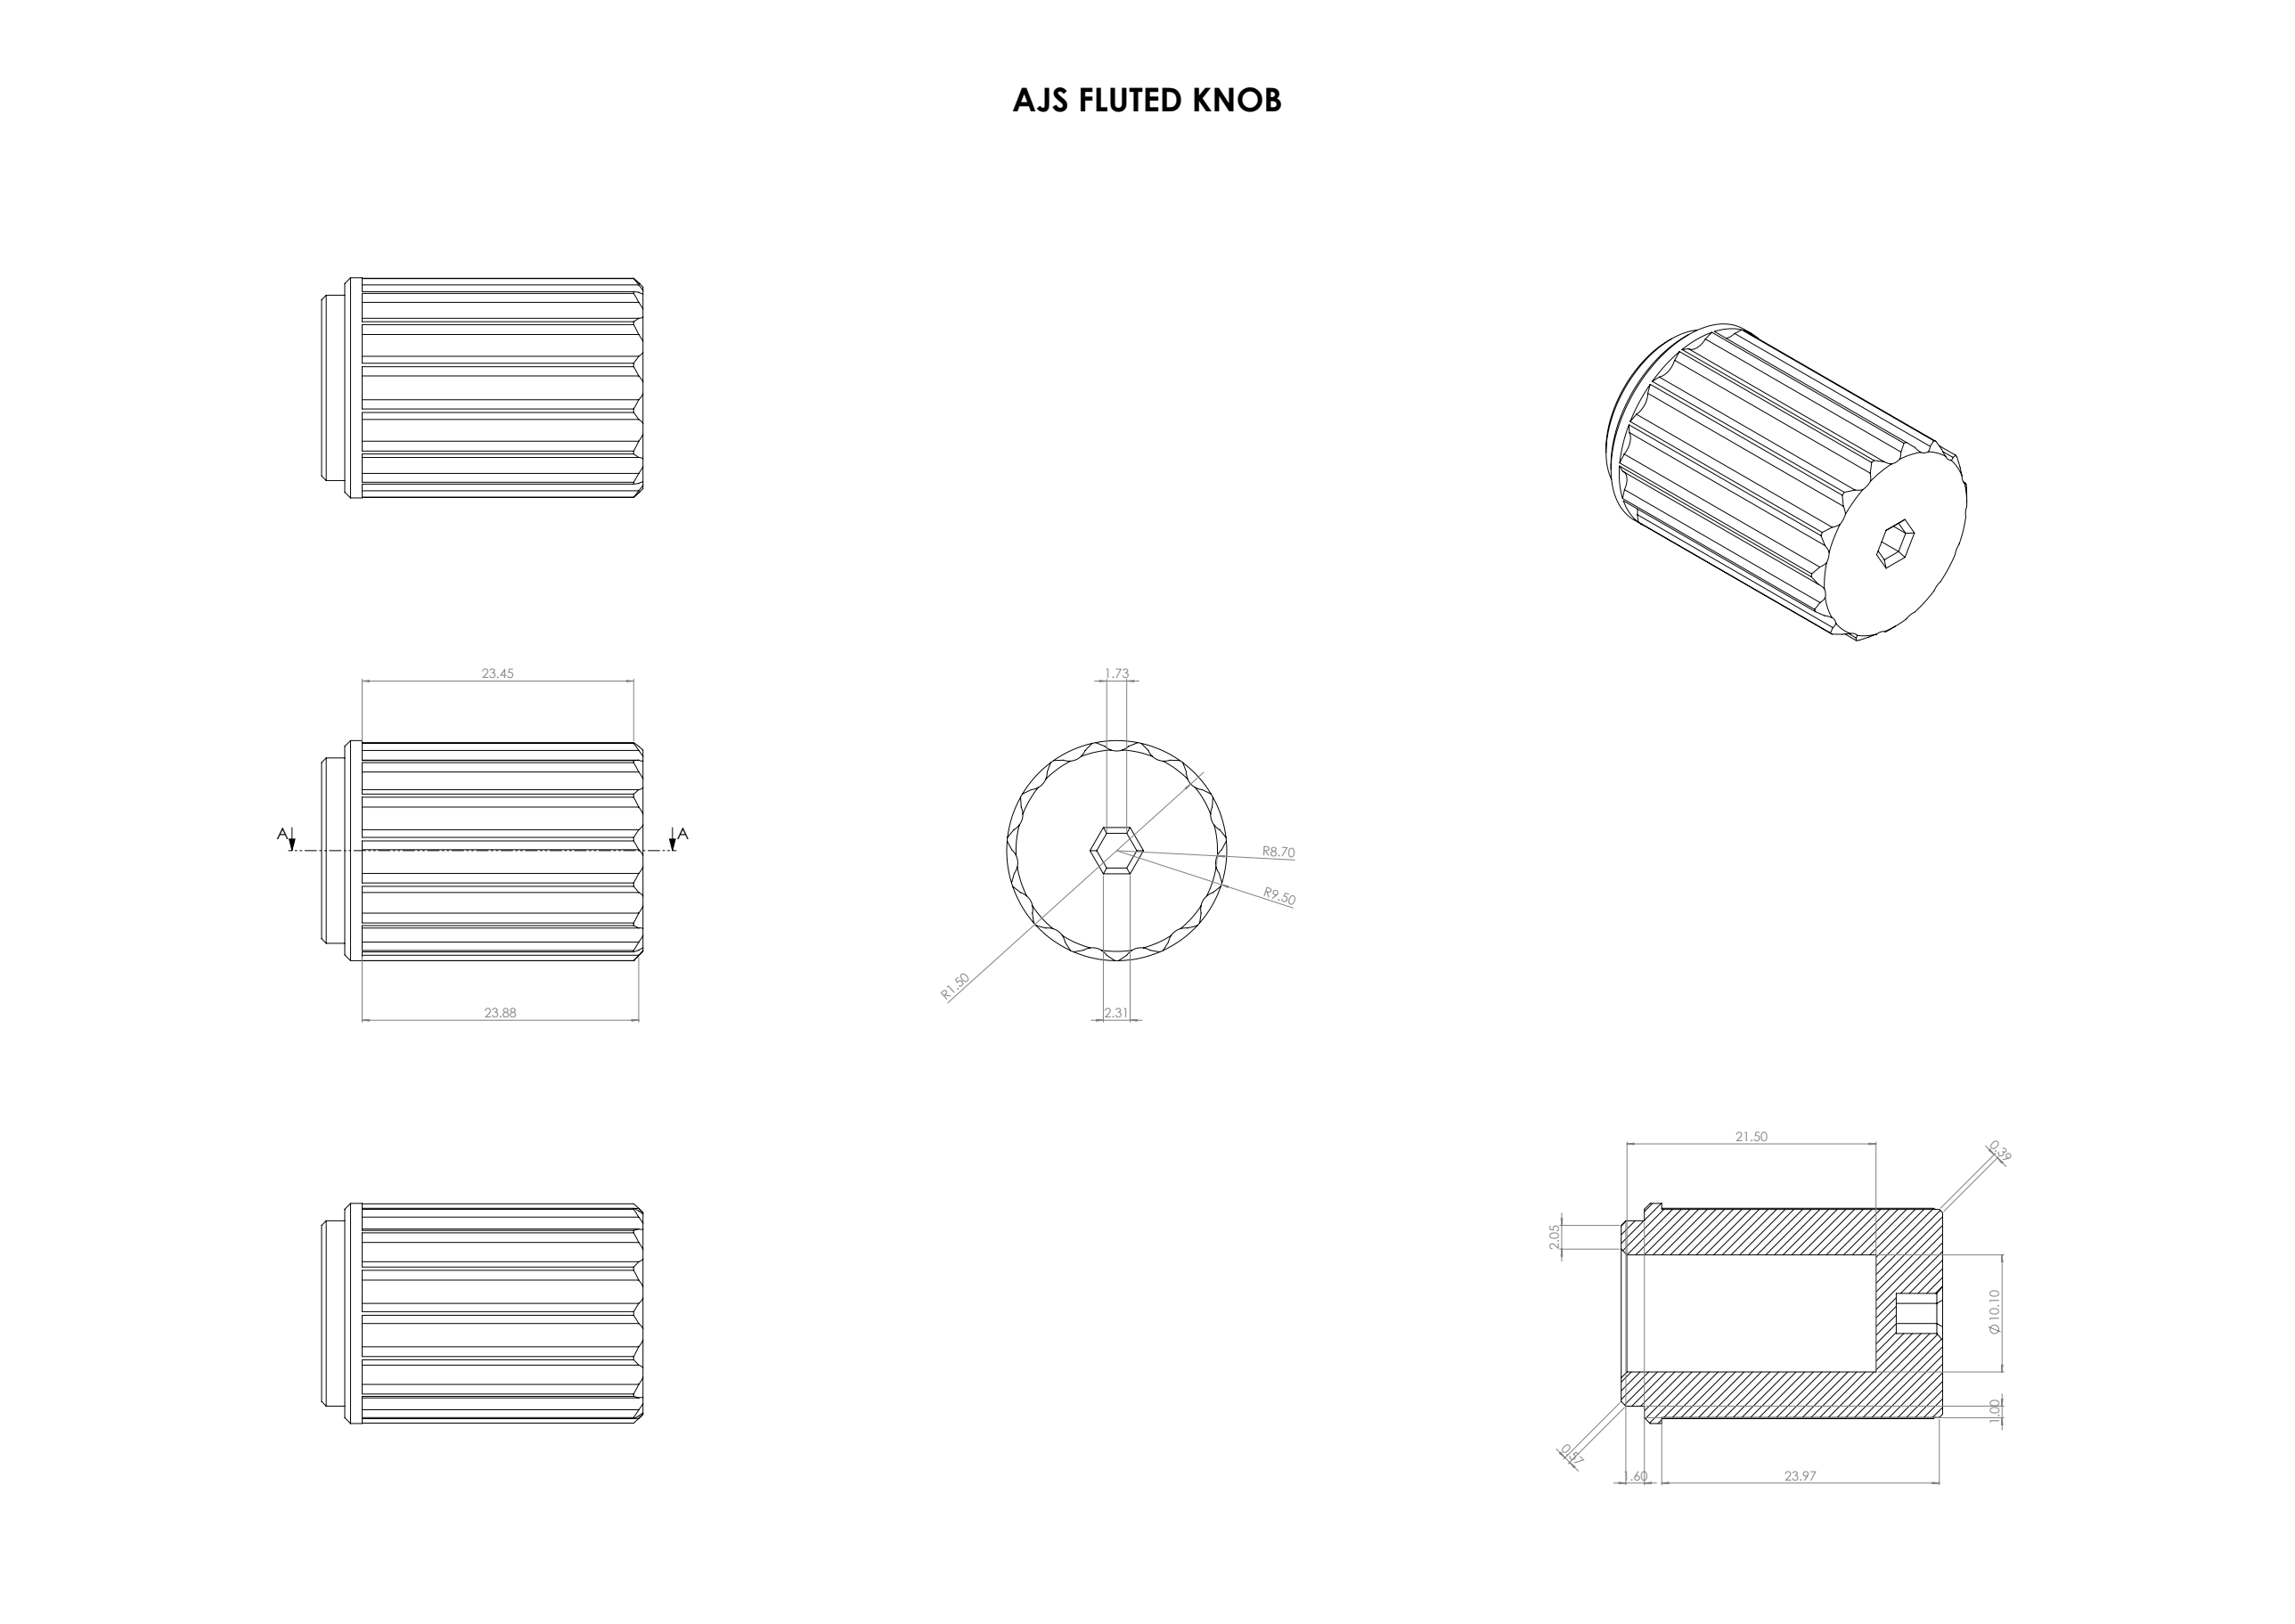
ISO-10303-21;
HEADER;
/* Generated by software containing ST-Developer
 * from STEP Tools, Inc. (www.steptools.com) 
 */

FILE_DESCRIPTION(
/* description */ (''),
/* implementation_level */ '2;1');

FILE_NAME(
/* name */ '06_AJS_Fluted_Knob.step',
/* time_stamp */ '2026-10-21T01:56:51-07:00',
/* author */ (''),
/* organization */ (''),
/* preprocessor_version */ 'ST-DEVELOPER v20.2',
/* originating_system */ 'Autodesk Translation Framework v15.15.0.0',
/* authorisation */ '');

FILE_SCHEMA (('AUTOMOTIVE_DESIGN { 1 0 10303 214 3 1 1 }'));
ENDSEC;

DATA;
#10=MECHANICAL_DESIGN_GEOMETRIC_PRESENTATION_REPRESENTATION('',(#287),#82384);
#202=(
BOUNDED_CURVE()
B_SPLINE_CURVE(2,(#80282,#80283,#80284),.UNSPECIFIED.,.F.,.F.)
B_SPLINE_CURVE_WITH_KNOTS((3,3),(0.095709435566232,0.188213402372322),
 .UNSPECIFIED.)
CURVE()
GEOMETRIC_REPRESENTATION_ITEM()
RATIONAL_B_SPLINE_CURVE((1.00220608042206,1.00217204690889,1.00001144171476))
REPRESENTATION_ITEM('')
);
#203=(
BOUNDED_CURVE()
B_SPLINE_CURVE(2,(#80312,#80313,#80314),.UNSPECIFIED.,.F.,.F.)
B_SPLINE_CURVE_WITH_KNOTS((3,3),(0.000244613971281809,0.0927485807773717),
 .UNSPECIFIED.)
CURVE()
GEOMETRIC_REPRESENTATION_ITEM()
RATIONAL_B_SPLINE_CURVE((1.00001144171476,1.00217204690889,1.00220608042206))
REPRESENTATION_ITEM('')
);
#204=(
BOUNDED_CURVE()
B_SPLINE_CURVE(2,(#80322,#80323,#80324),.UNSPECIFIED.,.F.,.F.)
B_SPLINE_CURVE_WITH_KNOTS((3,3),(0.0957094355662357,0.188213402372324),
 .UNSPECIFIED.)
CURVE()
GEOMETRIC_REPRESENTATION_ITEM()
RATIONAL_B_SPLINE_CURVE((1.00220608042216,1.00217204690899,1.00001144171476))
REPRESENTATION_ITEM('')
);
#205=(
BOUNDED_CURVE()
B_SPLINE_CURVE(2,(#80469,#80470,#80471),.UNSPECIFIED.,.F.,.F.)
B_SPLINE_CURVE_WITH_KNOTS((3,3),(0.000244613971281676,0.0927485807773712),
 .UNSPECIFIED.)
CURVE()
GEOMETRIC_REPRESENTATION_ITEM()
RATIONAL_B_SPLINE_CURVE((1.00001144171476,1.00217204690889,1.00220608042206))
REPRESENTATION_ITEM('')
);
#206=(
BOUNDED_CURVE()
B_SPLINE_CURVE(2,(#80475,#80476,#80477),.UNSPECIFIED.,.F.,.F.)
B_SPLINE_CURVE_WITH_KNOTS((3,3),(0.0957094355662342,0.188213402372322),
 .UNSPECIFIED.)
CURVE()
GEOMETRIC_REPRESENTATION_ITEM()
RATIONAL_B_SPLINE_CURVE((1.00220608042205,1.00217204690887,1.00001144171476))
REPRESENTATION_ITEM('')
);
#207=(
BOUNDED_CURVE()
B_SPLINE_CURVE(2,(#80504,#80505,#80506),.UNSPECIFIED.,.F.,.F.)
B_SPLINE_CURVE_WITH_KNOTS((3,3),(0.000244613971281263,0.0927485807773676),
 .UNSPECIFIED.)
CURVE()
GEOMETRIC_REPRESENTATION_ITEM()
RATIONAL_B_SPLINE_CURVE((1.00001144171476,1.00217204690908,1.00220608042225))
REPRESENTATION_ITEM('')
);
#208=(
BOUNDED_CURVE()
B_SPLINE_CURVE(2,(#80510,#80511,#80512),.UNSPECIFIED.,.F.,.F.)
B_SPLINE_CURVE_WITH_KNOTS((3,3),(0.0957094355662345,0.188213402372322),
 .UNSPECIFIED.)
CURVE()
GEOMETRIC_REPRESENTATION_ITEM()
RATIONAL_B_SPLINE_CURVE((1.00220608042216,1.00217204690899,1.00001144171476))
REPRESENTATION_ITEM('')
);
#209=(
BOUNDED_CURVE()
B_SPLINE_CURVE(2,(#80539,#80540,#80541),.UNSPECIFIED.,.F.,.F.)
B_SPLINE_CURVE_WITH_KNOTS((3,3),(0.000244613971281759,0.0927485807773703),
 .UNSPECIFIED.)
CURVE()
GEOMETRIC_REPRESENTATION_ITEM()
RATIONAL_B_SPLINE_CURVE((1.00001144171476,1.00217204690897,1.00220608042214))
REPRESENTATION_ITEM('')
);
#210=(
BOUNDED_CURVE()
B_SPLINE_CURVE(2,(#80545,#80546,#80547),.UNSPECIFIED.,.F.,.F.)
B_SPLINE_CURVE_WITH_KNOTS((3,3),(0.0957094355662337,0.188213402372321),
 .UNSPECIFIED.)
CURVE()
GEOMETRIC_REPRESENTATION_ITEM()
RATIONAL_B_SPLINE_CURVE((1.00220608042215,1.00217204690897,1.00001144171476))
REPRESENTATION_ITEM('')
);
#211=(
BOUNDED_CURVE()
B_SPLINE_CURVE(2,(#80574,#80575,#80576),.UNSPECIFIED.,.F.,.F.)
B_SPLINE_CURVE_WITH_KNOTS((3,3),(0.000244613971281829,0.0927485807773718),
 .UNSPECIFIED.)
CURVE()
GEOMETRIC_REPRESENTATION_ITEM()
RATIONAL_B_SPLINE_CURVE((1.00001144171476,1.00217204690888,1.00220608042205))
REPRESENTATION_ITEM('')
);
#212=(
BOUNDED_CURVE()
B_SPLINE_CURVE(2,(#80580,#80581,#80582),.UNSPECIFIED.,.F.,.F.)
B_SPLINE_CURVE_WITH_KNOTS((3,3),(0.0957094355662314,0.188213402372321),
 .UNSPECIFIED.)
CURVE()
GEOMETRIC_REPRESENTATION_ITEM()
RATIONAL_B_SPLINE_CURVE((1.00220608042206,1.00217204690889,1.00001144171476))
REPRESENTATION_ITEM('')
);
#213=(
BOUNDED_CURVE()
B_SPLINE_CURVE(2,(#80609,#80610,#80611),.UNSPECIFIED.,.F.,.F.)
B_SPLINE_CURVE_WITH_KNOTS((3,3),(0.000244613971281268,0.0927485807773693),
 .UNSPECIFIED.)
CURVE()
GEOMETRIC_REPRESENTATION_ITEM()
RATIONAL_B_SPLINE_CURVE((1.00001144171476,1.00217204690897,1.00220608042215))
REPRESENTATION_ITEM('')
);
#214=(
BOUNDED_CURVE()
B_SPLINE_CURVE(2,(#80615,#80616,#80617),.UNSPECIFIED.,.F.,.F.)
B_SPLINE_CURVE_WITH_KNOTS((3,3),(0.0957094355662326,0.188213402372321),
 .UNSPECIFIED.)
CURVE()
GEOMETRIC_REPRESENTATION_ITEM()
RATIONAL_B_SPLINE_CURVE((1.00220608042217,1.002172046909,1.00001144171476))
REPRESENTATION_ITEM('')
);
#215=(
BOUNDED_CURVE()
B_SPLINE_CURVE(2,(#80644,#80645,#80646),.UNSPECIFIED.,.F.,.F.)
B_SPLINE_CURVE_WITH_KNOTS((3,3),(0.000244613971283097,0.0927485807773713),
 .UNSPECIFIED.)
CURVE()
GEOMETRIC_REPRESENTATION_ITEM()
RATIONAL_B_SPLINE_CURVE((1.00001144171476,1.002172046909,1.00220608042218))
REPRESENTATION_ITEM('')
);
#216=(
BOUNDED_CURVE()
B_SPLINE_CURVE(2,(#80650,#80651,#80652),.UNSPECIFIED.,.F.,.F.)
B_SPLINE_CURVE_WITH_KNOTS((3,3),(0.0957094355662316,0.188213402372321),
 .UNSPECIFIED.)
CURVE()
GEOMETRIC_REPRESENTATION_ITEM()
RATIONAL_B_SPLINE_CURVE((1.00220608042227,1.00217204690909,1.00001144171476))
REPRESENTATION_ITEM('')
);
#217=(
BOUNDED_CURVE()
B_SPLINE_CURVE(2,(#80679,#80680,#80681),.UNSPECIFIED.,.F.,.F.)
B_SPLINE_CURVE_WITH_KNOTS((3,3),(0.000244613971281759,0.09274858077737),
 .UNSPECIFIED.)
CURVE()
GEOMETRIC_REPRESENTATION_ITEM()
RATIONAL_B_SPLINE_CURVE((1.00001144171476,1.00217204690888,1.00220608042205))
REPRESENTATION_ITEM('')
);
#218=(
BOUNDED_CURVE()
B_SPLINE_CURVE(2,(#80685,#80686,#80687),.UNSPECIFIED.,.F.,.F.)
B_SPLINE_CURVE_WITH_KNOTS((3,3),(0.0957094355662316,0.18821340237232),
 .UNSPECIFIED.)
CURVE()
GEOMETRIC_REPRESENTATION_ITEM()
RATIONAL_B_SPLINE_CURVE((1.00220608042213,1.00217204690896,1.00001144171476))
REPRESENTATION_ITEM('')
);
#219=(
BOUNDED_CURVE()
B_SPLINE_CURVE(2,(#80714,#80715,#80716),.UNSPECIFIED.,.F.,.F.)
B_SPLINE_CURVE_WITH_KNOTS((3,3),(0.000244613971281648,0.0927485807773707),
 .UNSPECIFIED.)
CURVE()
GEOMETRIC_REPRESENTATION_ITEM()
RATIONAL_B_SPLINE_CURVE((1.00001144171476,1.00217204690889,1.00220608042206))
REPRESENTATION_ITEM('')
);
#220=(
BOUNDED_CURVE()
B_SPLINE_CURVE(2,(#80720,#80721,#80722),.UNSPECIFIED.,.F.,.F.)
B_SPLINE_CURVE_WITH_KNOTS((3,3),(0.0957094355662329,0.188213402372321),
 .UNSPECIFIED.)
CURVE()
GEOMETRIC_REPRESENTATION_ITEM()
RATIONAL_B_SPLINE_CURVE((1.00220608042214,1.00217204690897,1.00001144171476))
REPRESENTATION_ITEM('')
);
#221=(
BOUNDED_CURVE()
B_SPLINE_CURVE(2,(#80749,#80750,#80751),.UNSPECIFIED.,.F.,.F.)
B_SPLINE_CURVE_WITH_KNOTS((3,3),(0.000244613971281549,0.0927485807773708),
 .UNSPECIFIED.)
CURVE()
GEOMETRIC_REPRESENTATION_ITEM()
RATIONAL_B_SPLINE_CURVE((1.00001144171476,1.002172046909,1.00220608042218))
REPRESENTATION_ITEM('')
);
#222=(
BOUNDED_CURVE()
B_SPLINE_CURVE(2,(#80755,#80756,#80757),.UNSPECIFIED.,.F.,.F.)
B_SPLINE_CURVE_WITH_KNOTS((3,3),(0.0957094355662331,0.188213402372322),
 .UNSPECIFIED.)
CURVE()
GEOMETRIC_REPRESENTATION_ITEM()
RATIONAL_B_SPLINE_CURVE((1.00220608042225,1.00217204690908,1.00001144171476))
REPRESENTATION_ITEM('')
);
#223=(
BOUNDED_CURVE()
B_SPLINE_CURVE(2,(#80784,#80785,#80786),.UNSPECIFIED.,.F.,.F.)
B_SPLINE_CURVE_WITH_KNOTS((3,3),(0.000244613971281458,0.0927485807773696),
 .UNSPECIFIED.)
CURVE()
GEOMETRIC_REPRESENTATION_ITEM()
RATIONAL_B_SPLINE_CURVE((1.00001144171476,1.00217204690908,1.00220608042225))
REPRESENTATION_ITEM('')
);
#224=(
BOUNDED_CURVE()
B_SPLINE_CURVE(2,(#80790,#80791,#80792),.UNSPECIFIED.,.F.,.F.)
B_SPLINE_CURVE_WITH_KNOTS((3,3),(0.0957094355662337,0.188213402372322),
 .UNSPECIFIED.)
CURVE()
GEOMETRIC_REPRESENTATION_ITEM()
RATIONAL_B_SPLINE_CURVE((1.00220608042226,1.00217204690909,1.00001144171476))
REPRESENTATION_ITEM('')
);
#225=(
BOUNDED_CURVE()
B_SPLINE_CURVE(2,(#80819,#80820,#80821),.UNSPECIFIED.,.F.,.F.)
B_SPLINE_CURVE_WITH_KNOTS((3,3),(0.000244613971281769,0.0927485807773717),
 .UNSPECIFIED.)
CURVE()
GEOMETRIC_REPRESENTATION_ITEM()
RATIONAL_B_SPLINE_CURVE((1.00001144171476,1.00217204690888,1.00220608042205))
REPRESENTATION_ITEM('')
);
#226=(
BOUNDED_CURVE()
B_SPLINE_CURVE(2,(#80825,#80826,#80827),.UNSPECIFIED.,.F.,.F.)
B_SPLINE_CURVE_WITH_KNOTS((3,3),(0.0957094355662335,0.188213402372321),
 .UNSPECIFIED.)
CURVE()
GEOMETRIC_REPRESENTATION_ITEM()
RATIONAL_B_SPLINE_CURVE((1.00220608042207,1.0021720469089,1.00001144171476))
REPRESENTATION_ITEM('')
);
#227=(
BOUNDED_CURVE()
B_SPLINE_CURVE(2,(#80854,#80855,#80856),.UNSPECIFIED.,.F.,.F.)
B_SPLINE_CURVE_WITH_KNOTS((3,3),(0.00024461397128167,0.0927485807773707),
 .UNSPECIFIED.)
CURVE()
GEOMETRIC_REPRESENTATION_ITEM()
RATIONAL_B_SPLINE_CURVE((1.00001144171476,1.00217204690889,1.00220608042207))
REPRESENTATION_ITEM('')
);
#228=(
BOUNDED_CURVE()
B_SPLINE_CURVE(2,(#80860,#80861,#80862),.UNSPECIFIED.,.F.,.F.)
B_SPLINE_CURVE_WITH_KNOTS((3,3),(0.0957094355662347,0.188213402372323),
 .UNSPECIFIED.)
CURVE()
GEOMETRIC_REPRESENTATION_ITEM()
RATIONAL_B_SPLINE_CURVE((1.00220608042226,1.00217204690908,1.00001144171476))
REPRESENTATION_ITEM('')
);
#229=(
BOUNDED_CURVE()
B_SPLINE_CURVE(2,(#80889,#80890,#80891),.UNSPECIFIED.,.F.,.F.)
B_SPLINE_CURVE_WITH_KNOTS((3,3),(0.000244613971281467,0.0927485807773707),
 .UNSPECIFIED.)
CURVE()
GEOMETRIC_REPRESENTATION_ITEM()
RATIONAL_B_SPLINE_CURVE((1.00001144171476,1.00217204690889,1.00220608042206))
REPRESENTATION_ITEM('')
);
#230=(
BOUNDED_CURVE()
B_SPLINE_CURVE(2,(#80895,#80896,#80897),.UNSPECIFIED.,.F.,.F.)
B_SPLINE_CURVE_WITH_KNOTS((3,3),(0.0957094355662333,0.188213402372321),
 .UNSPECIFIED.)
CURVE()
GEOMETRIC_REPRESENTATION_ITEM()
RATIONAL_B_SPLINE_CURVE((1.00220608042207,1.00217204690889,1.00001144171476))
REPRESENTATION_ITEM('')
);
#231=(
BOUNDED_CURVE()
B_SPLINE_CURVE(2,(#80924,#80925,#80926),.UNSPECIFIED.,.F.,.F.)
B_SPLINE_CURVE_WITH_KNOTS((3,3),(0.000244613971281619,0.0927485807773719),
 .UNSPECIFIED.)
CURVE()
GEOMETRIC_REPRESENTATION_ITEM()
RATIONAL_B_SPLINE_CURVE((1.00001144171476,1.00217204690898,1.00220608042215))
REPRESENTATION_ITEM('')
);
#249=SHAPE_REPRESENTATION_RELATIONSHIP('SRR','None',#82483,#268);
#268=ADVANCED_BREP_SHAPE_REPRESENTATION('',(#306),#82382);
#287=STYLED_ITEM('',(#82624),#306);
#306=MANIFOLD_SOLID_BREP('Body1',#30678);
#1003=CYLINDRICAL_SURFACE('',#33159,5.05);
#1004=CYLINDRICAL_SURFACE('',#33164,1.5);
#1005=CYLINDRICAL_SURFACE('',#33171,9.5);
#1006=CYLINDRICAL_SURFACE('',#33204,1.5);
#1007=CYLINDRICAL_SURFACE('',#33211,1.5);
#1008=CYLINDRICAL_SURFACE('',#33218,1.5);
#1009=CYLINDRICAL_SURFACE('',#33225,1.5);
#1010=CYLINDRICAL_SURFACE('',#33232,1.5);
#1011=CYLINDRICAL_SURFACE('',#33239,1.5);
#1012=CYLINDRICAL_SURFACE('',#33246,1.5);
#1013=CYLINDRICAL_SURFACE('',#33253,1.5);
#1014=CYLINDRICAL_SURFACE('',#33260,1.5);
#1015=CYLINDRICAL_SURFACE('',#33267,1.5);
#1016=CYLINDRICAL_SURFACE('',#33274,1.5);
#1017=CYLINDRICAL_SURFACE('',#33281,1.5);
#1018=CYLINDRICAL_SURFACE('',#33288,1.5);
#1019=CYLINDRICAL_SURFACE('',#33295,1.5);
#1020=CYLINDRICAL_SURFACE('',#33332,8.);
#1777=CIRCLE('',#33156,5.55);
#1778=CIRCLE('',#33157,5.05);
#1779=CIRCLE('',#33158,5.05);
#1780=CIRCLE('',#33160,5.05);
#1781=CIRCLE('',#33162,7.6);
#1782=CIRCLE('',#33165,1.5);
#1783=CIRCLE('',#33166,1.5);
#1784=CIRCLE('',#33169,9.5);
#1785=CIRCLE('',#33170,8.7);
#1786=CIRCLE('',#33172,9.5);
#1787=CIRCLE('',#33173,9.5);
#1788=CIRCLE('',#33174,9.5);
#1789=CIRCLE('',#33175,9.5);
#1790=CIRCLE('',#33176,9.5);
#1791=CIRCLE('',#33177,9.5);
#1792=CIRCLE('',#33178,9.5);
#1793=CIRCLE('',#33179,9.5);
#1794=CIRCLE('',#33180,9.5);
#1795=CIRCLE('',#33181,9.5);
#1796=CIRCLE('',#33182,9.5);
#1797=CIRCLE('',#33183,9.5);
#1798=CIRCLE('',#33184,9.5);
#1799=CIRCLE('',#33185,9.5);
#1800=CIRCLE('',#33186,9.5);
#1801=CIRCLE('',#33187,9.5);
#1802=CIRCLE('',#33188,9.5);
#1803=CIRCLE('',#33189,9.5);
#1804=CIRCLE('',#33190,9.5);
#1805=CIRCLE('',#33191,9.5);
#1806=CIRCLE('',#33192,9.5);
#1807=CIRCLE('',#33193,9.5);
#1808=CIRCLE('',#33194,9.5);
#1809=CIRCLE('',#33195,9.5);
#1810=CIRCLE('',#33196,9.5);
#1811=CIRCLE('',#33197,9.5);
#1812=CIRCLE('',#33198,9.5);
#1813=CIRCLE('',#33199,9.5);
#1814=CIRCLE('',#33200,9.5);
#1815=CIRCLE('',#33201,9.5);
#1816=CIRCLE('',#33202,9.5);
#1817=CIRCLE('',#33205,1.5);
#1818=CIRCLE('',#33206,1.5);
#1819=CIRCLE('',#33209,8.7);
#1820=CIRCLE('',#33212,1.5);
#1821=CIRCLE('',#33213,1.5);
#1822=CIRCLE('',#33216,8.7);
#1823=CIRCLE('',#33219,1.5);
#1824=CIRCLE('',#33220,1.5);
#1825=CIRCLE('',#33223,8.7);
#1826=CIRCLE('',#33226,1.5);
#1827=CIRCLE('',#33227,1.5);
#1828=CIRCLE('',#33230,8.7);
#1829=CIRCLE('',#33233,1.5);
#1830=CIRCLE('',#33234,1.5);
#1831=CIRCLE('',#33237,8.7);
#1832=CIRCLE('',#33240,1.5);
#1833=CIRCLE('',#33241,1.5);
#1834=CIRCLE('',#33244,8.7);
#1835=CIRCLE('',#33247,1.5);
#1836=CIRCLE('',#33248,1.5);
#1837=CIRCLE('',#33251,8.7);
#1838=CIRCLE('',#33254,1.5);
#1839=CIRCLE('',#33255,1.5);
#1840=CIRCLE('',#33258,8.7);
#1841=CIRCLE('',#33261,1.5);
#1842=CIRCLE('',#33262,1.5);
#1843=CIRCLE('',#33265,8.7);
#1844=CIRCLE('',#33268,1.5);
#1845=CIRCLE('',#33269,1.5);
#1846=CIRCLE('',#33272,8.7);
#1847=CIRCLE('',#33275,1.5);
#1848=CIRCLE('',#33276,1.5);
#1849=CIRCLE('',#33279,8.7);
#1850=CIRCLE('',#33282,1.5);
#1851=CIRCLE('',#33283,1.5);
#1852=CIRCLE('',#33286,8.7);
#1853=CIRCLE('',#33289,1.5);
#1854=CIRCLE('',#33290,1.5);
#1855=CIRCLE('',#33293,8.7);
#1856=CIRCLE('',#33296,1.5);
#1857=CIRCLE('',#33297,1.5);
#1858=CIRCLE('',#33309,8.7);
#1859=CIRCLE('',#33331,8.);
#1860=CIRCLE('',#33333,8.);
#1861=CIRCLE('',#33335,9.);
#2063=CONICAL_SURFACE('',#33155,5.3,0.785398163397451);
#2064=CONICAL_SURFACE('',#33168,9.1,0.785398163397454);
#2065=CONICAL_SURFACE('',#33208,9.1,0.785398163397454);
#2066=CONICAL_SURFACE('',#33215,9.1,0.785398163397454);
#2067=CONICAL_SURFACE('',#33222,9.1,0.785398163397454);
#2068=CONICAL_SURFACE('',#33229,9.1,0.785398163397454);
#2069=CONICAL_SURFACE('',#33236,9.1,0.785398163397454);
#2070=CONICAL_SURFACE('',#33243,9.1,0.785398163397454);
#2071=CONICAL_SURFACE('',#33250,9.1,0.785398163397454);
#2072=CONICAL_SURFACE('',#33257,9.1,0.785398163397454);
#2073=CONICAL_SURFACE('',#33264,9.1,0.785398163397454);
#2074=CONICAL_SURFACE('',#33271,9.1,0.785398163397454);
#2075=CONICAL_SURFACE('',#33278,9.1,0.785398163397454);
#2076=CONICAL_SURFACE('',#33285,9.1,0.785398163397454);
#2077=CONICAL_SURFACE('',#33292,9.1,0.785398163397454);
#2078=CONICAL_SURFACE('',#33329,9.1,0.785398163397454);
#2079=CONICAL_SURFACE('',#33330,7.8,0.785398163397454);
#2080=CONICAL_SURFACE('',#33336,9.25,0.785398163397445);
#3220=B_SPLINE_CURVE_WITH_KNOTS('',3,(#80296,#80297,#80298,#80299,#80300,
#80301),.UNSPECIFIED.,.F.,.F.,(4,2,4),(0.300223039487565,0.349769627099692,
0.370274237441758),.UNSPECIFIED.);
#3221=B_SPLINE_CURVE_WITH_KNOTS('',3,(#80304,#80305,#80306,#80307,#80308,
#80309),.UNSPECIFIED.,.F.,.F.,(4,2,4),(0.128903119732732,0.149407730074798,
0.198954317686925),.UNSPECIFIED.);
#3222=B_SPLINE_CURVE_WITH_KNOTS('',3,(#80326,#80327,#80328,#80329,#80330,
#80331),.UNSPECIFIED.,.F.,.F.,(4,2,4),(0.128903119732731,0.149407730074798,
0.198954317686925),.UNSPECIFIED.);
#3223=B_SPLINE_CURVE_WITH_KNOTS('',3,(#80461,#80462,#80463,#80464,#80465,
#80466),.UNSPECIFIED.,.F.,.F.,(4,2,4),(0.300223039487565,0.349769627099692,
0.370274237441758),.UNSPECIFIED.);
#3224=B_SPLINE_CURVE_WITH_KNOTS('',3,(#80479,#80480,#80481,#80482,#80483,
#80484),.UNSPECIFIED.,.F.,.F.,(4,2,4),(0.128903119732732,0.149407730074798,
0.198954317686925),.UNSPECIFIED.);
#3225=B_SPLINE_CURVE_WITH_KNOTS('',3,(#80496,#80497,#80498,#80499,#80500,
#80501),.UNSPECIFIED.,.F.,.F.,(4,2,4),(0.300223039487565,0.349769627099692,
0.370274237441758),.UNSPECIFIED.);
#3226=B_SPLINE_CURVE_WITH_KNOTS('',3,(#80514,#80515,#80516,#80517,#80518,
#80519),.UNSPECIFIED.,.F.,.F.,(4,2,4),(0.128903119732732,0.149407730074798,
0.198954317686925),.UNSPECIFIED.);
#3227=B_SPLINE_CURVE_WITH_KNOTS('',3,(#80531,#80532,#80533,#80534,#80535,
#80536),.UNSPECIFIED.,.F.,.F.,(4,2,4),(0.300223039487565,0.349769627099692,
0.370274237441758),.UNSPECIFIED.);
#3228=B_SPLINE_CURVE_WITH_KNOTS('',3,(#80549,#80550,#80551,#80552,#80553,
#80554),.UNSPECIFIED.,.F.,.F.,(4,2,4),(0.128903119732731,0.149407730074798,
0.198954317686925),.UNSPECIFIED.);
#3229=B_SPLINE_CURVE_WITH_KNOTS('',3,(#80566,#80567,#80568,#80569,#80570,
#80571),.UNSPECIFIED.,.F.,.F.,(4,2,4),(0.300223039487565,0.349769627099692,
0.370274237441758),.UNSPECIFIED.);
#3230=B_SPLINE_CURVE_WITH_KNOTS('',3,(#80584,#80585,#80586,#80587,#80588,
#80589),.UNSPECIFIED.,.F.,.F.,(4,2,4),(0.128903119732732,0.149407730074798,
0.198954317686925),.UNSPECIFIED.);
#3231=B_SPLINE_CURVE_WITH_KNOTS('',3,(#80601,#80602,#80603,#80604,#80605,
#80606),.UNSPECIFIED.,.F.,.F.,(4,2,4),(0.300223039487565,0.349769627099692,
0.370274237441759),.UNSPECIFIED.);
#3232=B_SPLINE_CURVE_WITH_KNOTS('',3,(#80619,#80620,#80621,#80622,#80623,
#80624),.UNSPECIFIED.,.F.,.F.,(4,2,4),(0.128903119732732,0.149407730074798,
0.198954317686923),.UNSPECIFIED.);
#3233=B_SPLINE_CURVE_WITH_KNOTS('',3,(#80636,#80637,#80638,#80639,#80640,
#80641),.UNSPECIFIED.,.F.,.F.,(4,2,4),(0.300223039487567,0.349769627099692,
0.370274237441759),.UNSPECIFIED.);
#3234=B_SPLINE_CURVE_WITH_KNOTS('',3,(#80654,#80655,#80656,#80657,#80658,
#80659),.UNSPECIFIED.,.F.,.F.,(4,2,4),(0.128903119732731,0.149407730074798,
0.198954317686924),.UNSPECIFIED.);
#3235=B_SPLINE_CURVE_WITH_KNOTS('',3,(#80671,#80672,#80673,#80674,#80675,
#80676),.UNSPECIFIED.,.F.,.F.,(4,2,4),(0.300223039487565,0.349769627099692,
0.370274237441758),.UNSPECIFIED.);
#3236=B_SPLINE_CURVE_WITH_KNOTS('',3,(#80689,#80690,#80691,#80692,#80693,
#80694),.UNSPECIFIED.,.F.,.F.,(4,2,4),(0.128903119732731,0.149407730074798,
0.198954317686925),.UNSPECIFIED.);
#3237=B_SPLINE_CURVE_WITH_KNOTS('',3,(#80706,#80707,#80708,#80709,#80710,
#80711),.UNSPECIFIED.,.F.,.F.,(4,2,4),(0.300223039487565,0.349769627099692,
0.370274237441758),.UNSPECIFIED.);
#3238=B_SPLINE_CURVE_WITH_KNOTS('',3,(#80724,#80725,#80726,#80727,#80728,
#80729),.UNSPECIFIED.,.F.,.F.,(4,2,4),(0.128903119732732,0.149407730074798,
0.198954317686924),.UNSPECIFIED.);
#3239=B_SPLINE_CURVE_WITH_KNOTS('',3,(#80741,#80742,#80743,#80744,#80745,
#80746),.UNSPECIFIED.,.F.,.F.,(4,2,4),(0.300223039487566,0.349769627099693,
0.370274237441759),.UNSPECIFIED.);
#3240=B_SPLINE_CURVE_WITH_KNOTS('',3,(#80759,#80760,#80761,#80762,#80763,
#80764),.UNSPECIFIED.,.F.,.F.,(4,2,4),(0.128903119732732,0.149407730074798,
0.198954317686925),.UNSPECIFIED.);
#3241=B_SPLINE_CURVE_WITH_KNOTS('',3,(#80776,#80777,#80778,#80779,#80780,
#80781),.UNSPECIFIED.,.F.,.F.,(4,2,4),(0.300223039487566,0.349769627099693,
0.370274237441759),.UNSPECIFIED.);
#3242=B_SPLINE_CURVE_WITH_KNOTS('',3,(#80794,#80795,#80796,#80797,#80798,
#80799),.UNSPECIFIED.,.F.,.F.,(4,2,4),(0.128903119732731,0.149407730074797,
0.198954317686924),.UNSPECIFIED.);
#3243=B_SPLINE_CURVE_WITH_KNOTS('',3,(#80811,#80812,#80813,#80814,#80815,
#80816),.UNSPECIFIED.,.F.,.F.,(4,2,4),(0.300223039487565,0.349769627099692,
0.370274237441758),.UNSPECIFIED.);
#3244=B_SPLINE_CURVE_WITH_KNOTS('',3,(#80829,#80830,#80831,#80832,#80833,
#80834),.UNSPECIFIED.,.F.,.F.,(4,2,4),(0.128903119732732,0.149407730074798,
0.198954317686925),.UNSPECIFIED.);
#3245=B_SPLINE_CURVE_WITH_KNOTS('',3,(#80846,#80847,#80848,#80849,#80850,
#80851),.UNSPECIFIED.,.F.,.F.,(4,2,4),(0.300223039487565,0.349769627099692,
0.370274237441758),.UNSPECIFIED.);
#3246=B_SPLINE_CURVE_WITH_KNOTS('',3,(#80864,#80865,#80866,#80867,#80868,
#80869),.UNSPECIFIED.,.F.,.F.,(4,2,4),(0.128903119732731,0.149407730074798,
0.198954317686925),.UNSPECIFIED.);
#3247=B_SPLINE_CURVE_WITH_KNOTS('',3,(#80881,#80882,#80883,#80884,#80885,
#80886),.UNSPECIFIED.,.F.,.F.,(4,2,4),(0.300223039487565,0.349769627099692,
0.370274237441758),.UNSPECIFIED.);
#3248=B_SPLINE_CURVE_WITH_KNOTS('',3,(#80899,#80900,#80901,#80902,#80903,
#80904),.UNSPECIFIED.,.F.,.F.,(4,2,4),(0.128903119732731,0.149407730074798,
0.198954317686925),.UNSPECIFIED.);
#3249=B_SPLINE_CURVE_WITH_KNOTS('',3,(#80916,#80917,#80918,#80919,#80920,
#80921),.UNSPECIFIED.,.F.,.F.,(4,2,4),(0.300223039487565,0.349769627099692,
0.370274237441759),.UNSPECIFIED.);
#3573=FACE_BOUND('',#7253,.T.);
#3574=FACE_BOUND('',#7324,.T.);
#3575=FACE_BOUND('',#7348,.T.);
#5205=FACE_OUTER_BOUND('',#7250,.T.);
#5206=FACE_OUTER_BOUND('',#7251,.T.);
#5207=FACE_OUTER_BOUND('',#7252,.T.);
#5208=FACE_OUTER_BOUND('',#7254,.T.);
#5209=FACE_OUTER_BOUND('',#7255,.T.);
#5210=FACE_OUTER_BOUND('',#7256,.T.);
#5211=FACE_OUTER_BOUND('',#7257,.T.);
#5212=FACE_OUTER_BOUND('',#7258,.T.);
#5213=FACE_OUTER_BOUND('',#7259,.T.);
#5214=FACE_OUTER_BOUND('',#7260,.T.);
#5215=FACE_OUTER_BOUND('',#7261,.T.);
#5216=FACE_OUTER_BOUND('',#7262,.T.);
#5217=FACE_OUTER_BOUND('',#7263,.T.);
#5218=FACE_OUTER_BOUND('',#7264,.T.);
#5219=FACE_OUTER_BOUND('',#7265,.T.);
#5220=FACE_OUTER_BOUND('',#7266,.T.);
#5221=FACE_OUTER_BOUND('',#7267,.T.);
#5222=FACE_OUTER_BOUND('',#7268,.T.);
#5223=FACE_OUTER_BOUND('',#7269,.T.);
#5224=FACE_OUTER_BOUND('',#7270,.T.);
#5225=FACE_OUTER_BOUND('',#7271,.T.);
#5226=FACE_OUTER_BOUND('',#7272,.T.);
#5227=FACE_OUTER_BOUND('',#7273,.T.);
#5228=FACE_OUTER_BOUND('',#7274,.T.);
#5229=FACE_OUTER_BOUND('',#7275,.T.);
#5230=FACE_OUTER_BOUND('',#7276,.T.);
#5231=FACE_OUTER_BOUND('',#7277,.T.);
#5232=FACE_OUTER_BOUND('',#7278,.T.);
#5233=FACE_OUTER_BOUND('',#7279,.T.);
#5234=FACE_OUTER_BOUND('',#7280,.T.);
#5235=FACE_OUTER_BOUND('',#7281,.T.);
#5236=FACE_OUTER_BOUND('',#7282,.T.);
#5237=FACE_OUTER_BOUND('',#7283,.T.);
#5238=FACE_OUTER_BOUND('',#7284,.T.);
#5239=FACE_OUTER_BOUND('',#7285,.T.);
#5240=FACE_OUTER_BOUND('',#7286,.T.);
#5241=FACE_OUTER_BOUND('',#7287,.T.);
#5242=FACE_OUTER_BOUND('',#7288,.T.);
#5243=FACE_OUTER_BOUND('',#7289,.T.);
#5244=FACE_OUTER_BOUND('',#7290,.T.);
#5245=FACE_OUTER_BOUND('',#7291,.T.);
#5246=FACE_OUTER_BOUND('',#7292,.T.);
#5247=FACE_OUTER_BOUND('',#7293,.T.);
#5248=FACE_OUTER_BOUND('',#7294,.T.);
#5249=FACE_OUTER_BOUND('',#7295,.T.);
#5250=FACE_OUTER_BOUND('',#7296,.T.);
#5251=FACE_OUTER_BOUND('',#7297,.T.);
#5252=FACE_OUTER_BOUND('',#7298,.T.);
#5253=FACE_OUTER_BOUND('',#7299,.T.);
#5254=FACE_OUTER_BOUND('',#7300,.T.);
#5255=FACE_OUTER_BOUND('',#7301,.T.);
#5256=FACE_OUTER_BOUND('',#7302,.T.);
#5257=FACE_OUTER_BOUND('',#7303,.T.);
#5258=FACE_OUTER_BOUND('',#7304,.T.);
#5259=FACE_OUTER_BOUND('',#7305,.T.);
#5260=FACE_OUTER_BOUND('',#7306,.T.);
#5261=FACE_OUTER_BOUND('',#7307,.T.);
#5262=FACE_OUTER_BOUND('',#7308,.T.);
#5263=FACE_OUTER_BOUND('',#7309,.T.);
#5264=FACE_OUTER_BOUND('',#7310,.T.);
#5265=FACE_OUTER_BOUND('',#7311,.T.);
#5266=FACE_OUTER_BOUND('',#7312,.T.);
#5267=FACE_OUTER_BOUND('',#7313,.T.);
#5268=FACE_OUTER_BOUND('',#7314,.T.);
#5269=FACE_OUTER_BOUND('',#7315,.T.);
#5270=FACE_OUTER_BOUND('',#7316,.T.);
#5271=FACE_OUTER_BOUND('',#7317,.T.);
#5272=FACE_OUTER_BOUND('',#7318,.T.);
#5273=FACE_OUTER_BOUND('',#7319,.T.);
#5274=FACE_OUTER_BOUND('',#7320,.T.);
#5275=FACE_OUTER_BOUND('',#7321,.T.);
#5276=FACE_OUTER_BOUND('',#7322,.T.);
#5277=FACE_OUTER_BOUND('',#7323,.T.);
#5278=FACE_OUTER_BOUND('',#7325,.T.);
#5279=FACE_OUTER_BOUND('',#7326,.T.);
#5280=FACE_OUTER_BOUND('',#7327,.T.);
#5281=FACE_OUTER_BOUND('',#7328,.T.);
#5282=FACE_OUTER_BOUND('',#7329,.T.);
#5283=FACE_OUTER_BOUND('',#7330,.T.);
#5284=FACE_OUTER_BOUND('',#7331,.T.);
#5285=FACE_OUTER_BOUND('',#7332,.T.);
#5286=FACE_OUTER_BOUND('',#7333,.T.);
#5287=FACE_OUTER_BOUND('',#7334,.T.);
#5288=FACE_OUTER_BOUND('',#7335,.T.);
#5289=FACE_OUTER_BOUND('',#7336,.T.);
#5290=FACE_OUTER_BOUND('',#7337,.T.);
#5291=FACE_OUTER_BOUND('',#7338,.T.);
#5292=FACE_OUTER_BOUND('',#7339,.T.);
#5293=FACE_OUTER_BOUND('',#7340,.T.);
#5294=FACE_OUTER_BOUND('',#7341,.T.);
#5295=FACE_OUTER_BOUND('',#7342,.T.);
#5296=FACE_OUTER_BOUND('',#7343,.T.);
#5297=FACE_OUTER_BOUND('',#7344,.T.);
#5298=FACE_OUTER_BOUND('',#7345,.T.);
#5299=FACE_OUTER_BOUND('',#7346,.T.);
#5300=FACE_OUTER_BOUND('',#7347,.T.);
#5301=FACE_OUTER_BOUND('',#7349,.T.);
#5302=FACE_OUTER_BOUND('',#7350,.T.);
#7250=EDGE_LOOP('',(#27399,#27400,#27401,#27402,#27403));
#7251=EDGE_LOOP('',(#27404,#27405,#27406,#27407,#27408));
#7252=EDGE_LOOP('',(#27409));
#7253=EDGE_LOOP('',(#27410));
#7254=EDGE_LOOP('',(#27411,#27412,#27413,#27414));
#7255=EDGE_LOOP('',(#27415,#27416,#27417,#27418,#27419,#27420));
#7256=EDGE_LOOP('',(#27421,#27422,#27423,#27424));
#7257=EDGE_LOOP('',(#27425,#27426,#27427,#27428,#27429,#27430));
#7258=EDGE_LOOP('',(#27431,#27432,#27433,#27434,#27435,#27436,#27437,#27438,
#27439,#27440,#27441,#27442,#27443,#27444,#27445,#27446,#27447,#27448,#27449,
#27450,#27451,#27452,#27453,#27454,#27455,#27456,#27457,#27458,#27459,#27460,
#27461,#27462,#27463,#27464,#27465,#27466,#27467,#27468,#27469,#27470,#27471,
#27472,#27473,#27474,#27475,#27476,#27477,#27478,#27479,#27480,#27481,#27482,
#27483,#27484,#27485,#27486,#27487,#27488,#27489,#27490,#27491,#27492,#27493,
#27494));
#7259=EDGE_LOOP('',(#27495,#27496,#27497,#27498));
#7260=EDGE_LOOP('',(#27499,#27500,#27501,#27502,#27503,#27504));
#7261=EDGE_LOOP('',(#27505,#27506,#27507,#27508));
#7262=EDGE_LOOP('',(#27509,#27510,#27511,#27512,#27513,#27514));
#7263=EDGE_LOOP('',(#27515,#27516,#27517,#27518));
#7264=EDGE_LOOP('',(#27519,#27520,#27521,#27522,#27523,#27524));
#7265=EDGE_LOOP('',(#27525,#27526,#27527,#27528));
#7266=EDGE_LOOP('',(#27529,#27530,#27531,#27532,#27533,#27534));
#7267=EDGE_LOOP('',(#27535,#27536,#27537,#27538));
#7268=EDGE_LOOP('',(#27539,#27540,#27541,#27542,#27543,#27544));
#7269=EDGE_LOOP('',(#27545,#27546,#27547,#27548));
#7270=EDGE_LOOP('',(#27549,#27550,#27551,#27552,#27553,#27554));
#7271=EDGE_LOOP('',(#27555,#27556,#27557,#27558));
#7272=EDGE_LOOP('',(#27559,#27560,#27561,#27562,#27563,#27564));
#7273=EDGE_LOOP('',(#27565,#27566,#27567,#27568));
#7274=EDGE_LOOP('',(#27569,#27570,#27571,#27572,#27573,#27574));
#7275=EDGE_LOOP('',(#27575,#27576,#27577,#27578));
#7276=EDGE_LOOP('',(#27579,#27580,#27581,#27582,#27583,#27584));
#7277=EDGE_LOOP('',(#27585,#27586,#27587,#27588));
#7278=EDGE_LOOP('',(#27589,#27590,#27591,#27592,#27593,#27594));
#7279=EDGE_LOOP('',(#27595,#27596,#27597,#27598));
#7280=EDGE_LOOP('',(#27599,#27600,#27601,#27602,#27603,#27604));
#7281=EDGE_LOOP('',(#27605,#27606,#27607,#27608));
#7282=EDGE_LOOP('',(#27609,#27610,#27611,#27612,#27613,#27614));
#7283=EDGE_LOOP('',(#27615,#27616,#27617,#27618));
#7284=EDGE_LOOP('',(#27619,#27620,#27621,#27622,#27623,#27624));
#7285=EDGE_LOOP('',(#27625,#27626,#27627,#27628));
#7286=EDGE_LOOP('',(#27629,#27630,#27631,#27632,#27633,#27634,#27635));
#7287=EDGE_LOOP('',(#27636,#27637,#27638,#27639));
#7288=EDGE_LOOP('',(#27640,#27641,#27642,#27643,#27644,#27645));
#7289=EDGE_LOOP('',(#27646,#27647,#27648,#27649));
#7290=EDGE_LOOP('',(#27650,#27651,#27652,#27653,#27654,#27655));
#7291=EDGE_LOOP('',(#27656,#27657,#27658,#27659));
#7292=EDGE_LOOP('',(#27660,#27661,#27662,#27663,#27664,#27665));
#7293=EDGE_LOOP('',(#27666,#27667,#27668,#27669));
#7294=EDGE_LOOP('',(#27670,#27671,#27672,#27673,#27674,#27675));
#7295=EDGE_LOOP('',(#27676,#27677,#27678,#27679));
#7296=EDGE_LOOP('',(#27680,#27681,#27682,#27683,#27684,#27685));
#7297=EDGE_LOOP('',(#27686,#27687,#27688,#27689));
#7298=EDGE_LOOP('',(#27690,#27691,#27692,#27693,#27694,#27695));
#7299=EDGE_LOOP('',(#27696,#27697,#27698,#27699));
#7300=EDGE_LOOP('',(#27700,#27701,#27702,#27703,#27704,#27705));
#7301=EDGE_LOOP('',(#27706,#27707,#27708,#27709));
#7302=EDGE_LOOP('',(#27710,#27711,#27712,#27713,#27714,#27715));
#7303=EDGE_LOOP('',(#27716,#27717,#27718,#27719));
#7304=EDGE_LOOP('',(#27720,#27721,#27722,#27723,#27724,#27725));
#7305=EDGE_LOOP('',(#27726,#27727,#27728,#27729));
#7306=EDGE_LOOP('',(#27730,#27731,#27732,#27733,#27734,#27735));
#7307=EDGE_LOOP('',(#27736,#27737,#27738,#27739));
#7308=EDGE_LOOP('',(#27740,#27741,#27742,#27743,#27744,#27745));
#7309=EDGE_LOOP('',(#27746,#27747,#27748,#27749));
#7310=EDGE_LOOP('',(#27750,#27751,#27752,#27753,#27754,#27755));
#7311=EDGE_LOOP('',(#27756,#27757,#27758,#27759));
#7312=EDGE_LOOP('',(#27760,#27761,#27762,#27763,#27764,#27765));
#7313=EDGE_LOOP('',(#27766,#27767,#27768,#27769));
#7314=EDGE_LOOP('',(#27770,#27771,#27772,#27773));
#7315=EDGE_LOOP('',(#27774,#27775,#27776,#27777));
#7316=EDGE_LOOP('',(#27778,#27779,#27780,#27781));
#7317=EDGE_LOOP('',(#27782,#27783,#27784,#27785));
#7318=EDGE_LOOP('',(#27786,#27787,#27788,#27789));
#7319=EDGE_LOOP('',(#27790,#27791,#27792,#27793));
#7320=EDGE_LOOP('',(#27794,#27795,#27796,#27797));
#7321=EDGE_LOOP('',(#27798,#27799,#27800,#27801));
#7322=EDGE_LOOP('',(#27802,#27803,#27804,#27805));
#7323=EDGE_LOOP('',(#27806,#27807,#27808,#27809,#27810,#27811,#27812,#27813,
#27814,#27815,#27816,#27817,#27818,#27819,#27820,#27821,#27822,#27823,#27824,
#27825,#27826,#27827,#27828,#27829,#27830,#27831,#27832,#27833,#27834,#27835));
#7324=EDGE_LOOP('',(#27836,#27837,#27838,#27839,#27840,#27841));
#7325=EDGE_LOOP('',(#27842,#27843,#27844,#27845));
#7326=EDGE_LOOP('',(#27846,#27847,#27848,#27849));
#7327=EDGE_LOOP('',(#27850,#27851,#27852,#27853));
#7328=EDGE_LOOP('',(#27854,#27855,#27856,#27857,#27858,#27859));
#7329=EDGE_LOOP('',(#27860,#27861,#27862,#27863));
#7330=EDGE_LOOP('',(#27864,#27865,#27866,#27867));
#7331=EDGE_LOOP('',(#27868,#27869,#27870,#27871));
#7332=EDGE_LOOP('',(#27872,#27873,#27874,#27875));
#7333=EDGE_LOOP('',(#27876,#27877,#27878,#27879));
#7334=EDGE_LOOP('',(#27880,#27881,#27882,#27883));
#7335=EDGE_LOOP('',(#27884,#27885,#27886,#27887));
#7336=EDGE_LOOP('',(#27888,#27889,#27890,#27891));
#7337=EDGE_LOOP('',(#27892,#27893,#27894,#27895));
#7338=EDGE_LOOP('',(#27896,#27897,#27898,#27899));
#7339=EDGE_LOOP('',(#27900,#27901,#27902,#27903));
#7340=EDGE_LOOP('',(#27904,#27905,#27906,#27907));
#7341=EDGE_LOOP('',(#27908,#27909,#27910,#27911));
#7342=EDGE_LOOP('',(#27912,#27913,#27914,#27915));
#7343=EDGE_LOOP('',(#27916,#27917,#27918,#27919));
#7344=EDGE_LOOP('',(#27920,#27921,#27922,#27923,#27924,#27925));
#7345=EDGE_LOOP('',(#27926,#27927,#27928,#27929));
#7346=EDGE_LOOP('',(#27930,#27931,#27932,#27933));
#7347=EDGE_LOOP('',(#27934));
#7348=EDGE_LOOP('',(#27935));
#7349=EDGE_LOOP('',(#27936,#27937,#27938,#27939));
#7350=EDGE_LOOP('',(#27940));
#9529=LINE('',#80268,#11835);
#9530=LINE('',#80275,#11836);
#9531=LINE('',#80286,#11837);
#9532=LINE('',#80288,#11838);
#9533=LINE('',#80289,#11839);
#9534=LINE('',#80294,#11840);
#9535=LINE('',#80316,#11841);
#9536=LINE('',#80317,#11842);
#9537=LINE('',#80337,#11843);
#9538=LINE('',#80341,#11844);
#9539=LINE('',#80345,#11845);
#9540=LINE('',#80349,#11846);
#9541=LINE('',#80353,#11847);
#9542=LINE('',#80357,#11848);
#9543=LINE('',#80361,#11849);
#9544=LINE('',#80365,#11850);
#9545=LINE('',#80369,#11851);
#9546=LINE('',#80373,#11852);
#9547=LINE('',#80377,#11853);
#9548=LINE('',#80381,#11854);
#9549=LINE('',#80385,#11855);
#9550=LINE('',#80389,#11856);
#9551=LINE('',#80393,#11857);
#9552=LINE('',#80398,#11858);
#9553=LINE('',#80402,#11859);
#9554=LINE('',#80406,#11860);
#9555=LINE('',#80410,#11861);
#9556=LINE('',#80414,#11862);
#9557=LINE('',#80418,#11863);
#9558=LINE('',#80422,#11864);
#9559=LINE('',#80426,#11865);
#9560=LINE('',#80430,#11866);
#9561=LINE('',#80434,#11867);
#9562=LINE('',#80438,#11868);
#9563=LINE('',#80442,#11869);
#9564=LINE('',#80446,#11870);
#9565=LINE('',#80449,#11871);
#9566=LINE('',#80453,#11872);
#9567=LINE('',#80454,#11873);
#9568=LINE('',#80459,#11874);
#9569=LINE('',#80472,#11875);
#9570=LINE('',#80488,#11876);
#9571=LINE('',#80489,#11877);
#9572=LINE('',#80494,#11878);
#9573=LINE('',#80507,#11879);
#9574=LINE('',#80523,#11880);
#9575=LINE('',#80524,#11881);
#9576=LINE('',#80529,#11882);
#9577=LINE('',#80542,#11883);
#9578=LINE('',#80558,#11884);
#9579=LINE('',#80559,#11885);
#9580=LINE('',#80564,#11886);
#9581=LINE('',#80577,#11887);
#9582=LINE('',#80593,#11888);
#9583=LINE('',#80594,#11889);
#9584=LINE('',#80599,#11890);
#9585=LINE('',#80612,#11891);
#9586=LINE('',#80628,#11892);
#9587=LINE('',#80629,#11893);
#9588=LINE('',#80634,#11894);
#9589=LINE('',#80647,#11895);
#9590=LINE('',#80663,#11896);
#9591=LINE('',#80664,#11897);
#9592=LINE('',#80669,#11898);
#9593=LINE('',#80682,#11899);
#9594=LINE('',#80698,#11900);
#9595=LINE('',#80699,#11901);
#9596=LINE('',#80704,#11902);
#9597=LINE('',#80717,#11903);
#9598=LINE('',#80733,#11904);
#9599=LINE('',#80734,#11905);
#9600=LINE('',#80739,#11906);
#9601=LINE('',#80752,#11907);
#9602=LINE('',#80768,#11908);
#9603=LINE('',#80769,#11909);
#9604=LINE('',#80774,#11910);
#9605=LINE('',#80787,#11911);
#9606=LINE('',#80803,#11912);
#9607=LINE('',#80804,#11913);
#9608=LINE('',#80809,#11914);
#9609=LINE('',#80822,#11915);
#9610=LINE('',#80838,#11916);
#9611=LINE('',#80839,#11917);
#9612=LINE('',#80844,#11918);
#9613=LINE('',#80857,#11919);
#9614=LINE('',#80873,#11920);
#9615=LINE('',#80874,#11921);
#9616=LINE('',#80879,#11922);
#9617=LINE('',#80892,#11923);
#9618=LINE('',#80908,#11924);
#9619=LINE('',#80909,#11925);
#9620=LINE('',#80914,#11926);
#9621=LINE('',#80927,#11927);
#9622=LINE('',#80931,#11928);
#9623=LINE('',#80933,#11929);
#9624=LINE('',#80935,#11930);
#9625=LINE('',#80936,#11931);
#9626=LINE('',#80939,#11932);
#9627=LINE('',#80941,#11933);
#9628=LINE('',#80942,#11934);
#9629=LINE('',#80946,#11935);
#9630=LINE('',#80948,#11936);
#9631=LINE('',#80950,#11937);
#9632=LINE('',#80951,#11938);
#9633=LINE('',#80954,#11939);
#9634=LINE('',#80956,#11940);
#9635=LINE('',#80957,#11941);
#9636=LINE('',#80959,#11942);
#9637=LINE('',#80960,#11943);
#9638=LINE('',#80962,#11944);
#9639=LINE('',#80963,#11945);
#9640=LINE('',#80966,#11946);
#9641=LINE('',#80968,#11947);
#9642=LINE('',#80969,#11948);
#9643=LINE('',#80972,#11949);
#9644=LINE('',#80973,#11950);
#9645=LINE('',#80976,#11951);
#9646=LINE('',#80977,#11952);
#9647=LINE('',#80982,#11953);
#9648=LINE('',#80983,#11954);
#9649=LINE('',#80986,#11955);
#9650=LINE('',#80987,#11956);
#9651=LINE('',#80989,#11957);
#9652=LINE('',#81010,#11958);
#9653=LINE('',#81014,#11959);
#9654=LINE('',#81019,#11960);
#11835=VECTOR('',#40094,5.3);
#11836=VECTOR('',#40103,5.05);
#11837=VECTOR('',#40110,10.);
#11838=VECTOR('',#40111,10.);
#11839=VECTOR('',#40112,10.);
#11840=VECTOR('',#40117,10.);
#11841=VECTOR('',#40122,10.);
#11842=VECTOR('',#40123,10.);
#11843=VECTOR('',#40134,10.);
#11844=VECTOR('',#40137,10.);
#11845=VECTOR('',#40140,10.);
#11846=VECTOR('',#40143,10.);
#11847=VECTOR('',#40146,10.);
#11848=VECTOR('',#40149,10.);
#11849=VECTOR('',#40152,10.);
#11850=VECTOR('',#40155,10.);
#11851=VECTOR('',#40158,10.);
#11852=VECTOR('',#40161,10.);
#11853=VECTOR('',#40164,10.);
#11854=VECTOR('',#40167,10.);
#11855=VECTOR('',#40170,10.);
#11856=VECTOR('',#40173,10.);
#11857=VECTOR('',#40176,9.5);
#11858=VECTOR('',#40181,10.);
#11859=VECTOR('',#40184,10.);
#11860=VECTOR('',#40187,10.);
#11861=VECTOR('',#40190,10.);
#11862=VECTOR('',#40193,10.);
#11863=VECTOR('',#40196,10.);
#11864=VECTOR('',#40199,10.);
#11865=VECTOR('',#40202,10.);
#11866=VECTOR('',#40205,10.);
#11867=VECTOR('',#40208,10.);
#11868=VECTOR('',#40211,10.);
#11869=VECTOR('',#40214,10.);
#11870=VECTOR('',#40217,10.);
#11871=VECTOR('',#40220,10.);
#11872=VECTOR('',#40225,10.);
#11873=VECTOR('',#40226,10.);
#11874=VECTOR('',#40231,10.);
#11875=VECTOR('',#40236,10.);
#11876=VECTOR('',#40243,10.);
#11877=VECTOR('',#40244,10.);
#11878=VECTOR('',#40249,10.);
#11879=VECTOR('',#40254,10.);
#11880=VECTOR('',#40261,10.);
#11881=VECTOR('',#40262,10.);
#11882=VECTOR('',#40267,10.);
#11883=VECTOR('',#40272,10.);
#11884=VECTOR('',#40279,10.);
#11885=VECTOR('',#40280,10.);
#11886=VECTOR('',#40285,10.);
#11887=VECTOR('',#40290,10.);
#11888=VECTOR('',#40297,10.);
#11889=VECTOR('',#40298,10.);
#11890=VECTOR('',#40303,10.);
#11891=VECTOR('',#40308,10.);
#11892=VECTOR('',#40315,10.);
#11893=VECTOR('',#40316,10.);
#11894=VECTOR('',#40321,10.);
#11895=VECTOR('',#40326,10.);
#11896=VECTOR('',#40333,10.);
#11897=VECTOR('',#40334,10.);
#11898=VECTOR('',#40339,10.);
#11899=VECTOR('',#40344,10.);
#11900=VECTOR('',#40351,10.);
#11901=VECTOR('',#40352,10.);
#11902=VECTOR('',#40357,10.);
#11903=VECTOR('',#40362,10.);
#11904=VECTOR('',#40369,10.);
#11905=VECTOR('',#40370,10.);
#11906=VECTOR('',#40375,10.);
#11907=VECTOR('',#40380,10.);
#11908=VECTOR('',#40387,10.);
#11909=VECTOR('',#40388,10.);
#11910=VECTOR('',#40393,10.);
#11911=VECTOR('',#40398,10.);
#11912=VECTOR('',#40405,10.);
#11913=VECTOR('',#40406,10.);
#11914=VECTOR('',#40411,10.);
#11915=VECTOR('',#40416,10.);
#11916=VECTOR('',#40423,10.);
#11917=VECTOR('',#40424,10.);
#11918=VECTOR('',#40429,10.);
#11919=VECTOR('',#40434,10.);
#11920=VECTOR('',#40441,10.);
#11921=VECTOR('',#40442,10.);
#11922=VECTOR('',#40447,10.);
#11923=VECTOR('',#40452,10.);
#11924=VECTOR('',#40459,10.);
#11925=VECTOR('',#40460,10.);
#11926=VECTOR('',#40465,10.);
#11927=VECTOR('',#40470,10.);
#11928=VECTOR('',#40473,10.);
#11929=VECTOR('',#40474,10.);
#11930=VECTOR('',#40475,10.);
#11931=VECTOR('',#40476,10.);
#11932=VECTOR('',#40479,10.);
#11933=VECTOR('',#40480,10.);
#11934=VECTOR('',#40481,10.);
#11935=VECTOR('',#40484,10.);
#11936=VECTOR('',#40485,10.);
#11937=VECTOR('',#40486,10.);
#11938=VECTOR('',#40487,10.);
#11939=VECTOR('',#40490,10.);
#11940=VECTOR('',#40491,10.);
#11941=VECTOR('',#40492,10.);
#11942=VECTOR('',#40495,10.);
#11943=VECTOR('',#40496,10.);
#11944=VECTOR('',#40499,10.);
#11945=VECTOR('',#40500,10.);
#11946=VECTOR('',#40503,10.);
#11947=VECTOR('',#40504,10.);
#11948=VECTOR('',#40505,10.);
#11949=VECTOR('',#40508,10.);
#11950=VECTOR('',#40509,10.);
#11951=VECTOR('',#40512,10.);
#11952=VECTOR('',#40513,10.);
#11953=VECTOR('',#40520,10.);
#11954=VECTOR('',#40521,10.);
#11955=VECTOR('',#40524,10.);
#11956=VECTOR('',#40525,10.);
#11957=VECTOR('',#40528,10.);
#11958=VECTOR('',#40567,7.8);
#11959=VECTOR('',#40572,8.);
#11960=VECTOR('',#40579,9.25);
#14628=VERTEX_POINT('',#80265);
#14629=VERTEX_POINT('',#80267);
#14630=VERTEX_POINT('',#80269);
#14631=VERTEX_POINT('',#80273);
#14632=VERTEX_POINT('',#80277);
#14633=VERTEX_POINT('',#80280);
#14634=VERTEX_POINT('',#80281);
#14635=VERTEX_POINT('',#80285);
#14636=VERTEX_POINT('',#80287);
#14637=VERTEX_POINT('',#80291);
#14638=VERTEX_POINT('',#80293);
#14639=VERTEX_POINT('',#80295);
#14640=VERTEX_POINT('',#80302);
#14641=VERTEX_POINT('',#80311);
#14642=VERTEX_POINT('',#80315);
#14643=VERTEX_POINT('',#80319);
#14644=VERTEX_POINT('',#80321);
#14645=VERTEX_POINT('',#80325);
#14646=VERTEX_POINT('',#80334);
#14647=VERTEX_POINT('',#80336);
#14648=VERTEX_POINT('',#80338);
#14649=VERTEX_POINT('',#80340);
#14650=VERTEX_POINT('',#80342);
#14651=VERTEX_POINT('',#80344);
#14652=VERTEX_POINT('',#80346);
#14653=VERTEX_POINT('',#80348);
#14654=VERTEX_POINT('',#80350);
#14655=VERTEX_POINT('',#80352);
#14656=VERTEX_POINT('',#80354);
#14657=VERTEX_POINT('',#80356);
#14658=VERTEX_POINT('',#80358);
#14659=VERTEX_POINT('',#80360);
#14660=VERTEX_POINT('',#80362);
#14661=VERTEX_POINT('',#80364);
#14662=VERTEX_POINT('',#80366);
#14663=VERTEX_POINT('',#80368);
#14664=VERTEX_POINT('',#80370);
#14665=VERTEX_POINT('',#80372);
#14666=VERTEX_POINT('',#80374);
#14667=VERTEX_POINT('',#80376);
#14668=VERTEX_POINT('',#80378);
#14669=VERTEX_POINT('',#80380);
#14670=VERTEX_POINT('',#80382);
#14671=VERTEX_POINT('',#80384);
#14672=VERTEX_POINT('',#80386);
#14673=VERTEX_POINT('',#80388);
#14674=VERTEX_POINT('',#80390);
#14675=VERTEX_POINT('',#80392);
#14676=VERTEX_POINT('',#80395);
#14677=VERTEX_POINT('',#80397);
#14678=VERTEX_POINT('',#80399);
#14679=VERTEX_POINT('',#80401);
#14680=VERTEX_POINT('',#80403);
#14681=VERTEX_POINT('',#80405);
#14682=VERTEX_POINT('',#80407);
#14683=VERTEX_POINT('',#80409);
#14684=VERTEX_POINT('',#80411);
#14685=VERTEX_POINT('',#80413);
#14686=VERTEX_POINT('',#80415);
#14687=VERTEX_POINT('',#80417);
#14688=VERTEX_POINT('',#80419);
#14689=VERTEX_POINT('',#80421);
#14690=VERTEX_POINT('',#80423);
#14691=VERTEX_POINT('',#80425);
#14692=VERTEX_POINT('',#80427);
#14693=VERTEX_POINT('',#80429);
#14694=VERTEX_POINT('',#80431);
#14695=VERTEX_POINT('',#80433);
#14696=VERTEX_POINT('',#80435);
#14697=VERTEX_POINT('',#80437);
#14698=VERTEX_POINT('',#80439);
#14699=VERTEX_POINT('',#80441);
#14700=VERTEX_POINT('',#80443);
#14701=VERTEX_POINT('',#80445);
#14702=VERTEX_POINT('',#80447);
#14703=VERTEX_POINT('',#80452);
#14704=VERTEX_POINT('',#80456);
#14705=VERTEX_POINT('',#80458);
#14706=VERTEX_POINT('',#80460);
#14707=VERTEX_POINT('',#80474);
#14708=VERTEX_POINT('',#80478);
#14709=VERTEX_POINT('',#80487);
#14710=VERTEX_POINT('',#80491);
#14711=VERTEX_POINT('',#80493);
#14712=VERTEX_POINT('',#80495);
#14713=VERTEX_POINT('',#80509);
#14714=VERTEX_POINT('',#80513);
#14715=VERTEX_POINT('',#80522);
#14716=VERTEX_POINT('',#80526);
#14717=VERTEX_POINT('',#80528);
#14718=VERTEX_POINT('',#80530);
#14719=VERTEX_POINT('',#80544);
#14720=VERTEX_POINT('',#80548);
#14721=VERTEX_POINT('',#80557);
#14722=VERTEX_POINT('',#80561);
#14723=VERTEX_POINT('',#80563);
#14724=VERTEX_POINT('',#80565);
#14725=VERTEX_POINT('',#80579);
#14726=VERTEX_POINT('',#80583);
#14727=VERTEX_POINT('',#80592);
#14728=VERTEX_POINT('',#80596);
#14729=VERTEX_POINT('',#80598);
#14730=VERTEX_POINT('',#80600);
#14731=VERTEX_POINT('',#80614);
#14732=VERTEX_POINT('',#80618);
#14733=VERTEX_POINT('',#80627);
#14734=VERTEX_POINT('',#80631);
#14735=VERTEX_POINT('',#80633);
#14736=VERTEX_POINT('',#80635);
#14737=VERTEX_POINT('',#80649);
#14738=VERTEX_POINT('',#80653);
#14739=VERTEX_POINT('',#80662);
#14740=VERTEX_POINT('',#80666);
#14741=VERTEX_POINT('',#80668);
#14742=VERTEX_POINT('',#80670);
#14743=VERTEX_POINT('',#80684);
#14744=VERTEX_POINT('',#80688);
#14745=VERTEX_POINT('',#80697);
#14746=VERTEX_POINT('',#80701);
#14747=VERTEX_POINT('',#80703);
#14748=VERTEX_POINT('',#80705);
#14749=VERTEX_POINT('',#80719);
#14750=VERTEX_POINT('',#80723);
#14751=VERTEX_POINT('',#80732);
#14752=VERTEX_POINT('',#80736);
#14753=VERTEX_POINT('',#80738);
#14754=VERTEX_POINT('',#80740);
#14755=VERTEX_POINT('',#80754);
#14756=VERTEX_POINT('',#80758);
#14757=VERTEX_POINT('',#80767);
#14758=VERTEX_POINT('',#80771);
#14759=VERTEX_POINT('',#80773);
#14760=VERTEX_POINT('',#80775);
#14761=VERTEX_POINT('',#80789);
#14762=VERTEX_POINT('',#80793);
#14763=VERTEX_POINT('',#80802);
#14764=VERTEX_POINT('',#80806);
#14765=VERTEX_POINT('',#80808);
#14766=VERTEX_POINT('',#80810);
#14767=VERTEX_POINT('',#80824);
#14768=VERTEX_POINT('',#80828);
#14769=VERTEX_POINT('',#80837);
#14770=VERTEX_POINT('',#80841);
#14771=VERTEX_POINT('',#80843);
#14772=VERTEX_POINT('',#80845);
#14773=VERTEX_POINT('',#80859);
#14774=VERTEX_POINT('',#80863);
#14775=VERTEX_POINT('',#80872);
#14776=VERTEX_POINT('',#80876);
#14777=VERTEX_POINT('',#80878);
#14778=VERTEX_POINT('',#80880);
#14779=VERTEX_POINT('',#80894);
#14780=VERTEX_POINT('',#80898);
#14781=VERTEX_POINT('',#80907);
#14782=VERTEX_POINT('',#80911);
#14783=VERTEX_POINT('',#80913);
#14784=VERTEX_POINT('',#80915);
#14785=VERTEX_POINT('',#80929);
#14786=VERTEX_POINT('',#80930);
#14787=VERTEX_POINT('',#80932);
#14788=VERTEX_POINT('',#80934);
#14789=VERTEX_POINT('',#80938);
#14790=VERTEX_POINT('',#80940);
#14791=VERTEX_POINT('',#80944);
#14792=VERTEX_POINT('',#80945);
#14793=VERTEX_POINT('',#80947);
#14794=VERTEX_POINT('',#80949);
#14795=VERTEX_POINT('',#80953);
#14796=VERTEX_POINT('',#80955);
#14797=VERTEX_POINT('',#80965);
#14798=VERTEX_POINT('',#80967);
#14799=VERTEX_POINT('',#80971);
#14800=VERTEX_POINT('',#80975);
#14801=VERTEX_POINT('',#80981);
#14802=VERTEX_POINT('',#80985);
#14803=VERTEX_POINT('',#81008);
#14804=VERTEX_POINT('',#81012);
#14805=VERTEX_POINT('',#81016);
#18921=EDGE_CURVE('',#14628,#14628,#1777,.T.);
#18922=EDGE_CURVE('',#14628,#14629,#9529,.T.);
#18923=EDGE_CURVE('',#14629,#14630,#1778,.T.);
#18924=EDGE_CURVE('',#14630,#14629,#1779,.T.);
#18925=EDGE_CURVE('',#14631,#14631,#1780,.T.);
#18926=EDGE_CURVE('',#14631,#14630,#9530,.T.);
#18927=EDGE_CURVE('',#14632,#14632,#1781,.T.);
#18928=EDGE_CURVE('',#14633,#14634,#202,.T.);
#18929=EDGE_CURVE('',#14634,#14635,#9531,.T.);
#18930=EDGE_CURVE('',#14635,#14636,#9532,.F.);
#18931=EDGE_CURVE('',#14636,#14633,#9533,.T.);
#18932=EDGE_CURVE('',#14637,#14636,#1782,.T.);
#18933=EDGE_CURVE('',#14638,#14637,#9534,.T.);
#18934=EDGE_CURVE('',#14639,#14638,#3220,.T.);
#18935=EDGE_CURVE('',#14640,#14639,#1783,.T.);
#18936=EDGE_CURVE('',#14633,#14640,#3221,.T.);
#18937=EDGE_CURVE('',#14641,#14638,#203,.T.);
#18938=EDGE_CURVE('',#14637,#14642,#9535,.F.);
#18939=EDGE_CURVE('',#14642,#14641,#9536,.T.);
#18940=EDGE_CURVE('',#14641,#14643,#1784,.T.);
#18941=EDGE_CURVE('',#14644,#14643,#204,.T.);
#18942=EDGE_CURVE('',#14644,#14645,#3222,.T.);
#18943=EDGE_CURVE('',#14639,#14645,#1785,.T.);
#18944=EDGE_CURVE('',#14646,#14634,#1786,.T.);
#18945=EDGE_CURVE('',#14647,#14646,#9537,.T.);
#18946=EDGE_CURVE('',#14647,#14648,#1787,.T.);
#18947=EDGE_CURVE('',#14649,#14648,#9538,.T.);
#18948=EDGE_CURVE('',#14650,#14649,#1788,.T.);
#18949=EDGE_CURVE('',#14651,#14650,#9539,.T.);
#18950=EDGE_CURVE('',#14651,#14652,#1789,.T.);
#18951=EDGE_CURVE('',#14653,#14652,#9540,.T.);
#18952=EDGE_CURVE('',#14654,#14653,#1790,.T.);
#18953=EDGE_CURVE('',#14655,#14654,#9541,.T.);
#18954=EDGE_CURVE('',#14655,#14656,#1791,.T.);
#18955=EDGE_CURVE('',#14657,#14656,#9542,.T.);
#18956=EDGE_CURVE('',#14658,#14657,#1792,.T.);
#18957=EDGE_CURVE('',#14659,#14658,#9543,.T.);
#18958=EDGE_CURVE('',#14659,#14660,#1793,.T.);
#18959=EDGE_CURVE('',#14661,#14660,#9544,.T.);
#18960=EDGE_CURVE('',#14662,#14661,#1794,.T.);
#18961=EDGE_CURVE('',#14663,#14662,#9545,.T.);
#18962=EDGE_CURVE('',#14663,#14664,#1795,.T.);
#18963=EDGE_CURVE('',#14665,#14664,#9546,.T.);
#18964=EDGE_CURVE('',#14666,#14665,#1796,.T.);
#18965=EDGE_CURVE('',#14667,#14666,#9547,.T.);
#18966=EDGE_CURVE('',#14667,#14668,#1797,.T.);
#18967=EDGE_CURVE('',#14669,#14668,#9548,.T.);
#18968=EDGE_CURVE('',#14670,#14669,#1798,.T.);
#18969=EDGE_CURVE('',#14671,#14670,#9549,.T.);
#18970=EDGE_CURVE('',#14671,#14672,#1799,.T.);
#18971=EDGE_CURVE('',#14673,#14672,#9550,.T.);
#18972=EDGE_CURVE('',#14674,#14673,#1800,.T.);
#18973=EDGE_CURVE('',#14674,#14675,#9551,.T.);
#18974=EDGE_CURVE('',#14675,#14675,#1801,.T.);
#18975=EDGE_CURVE('',#14676,#14674,#1802,.T.);
#18976=EDGE_CURVE('',#14677,#14676,#9552,.T.);
#18977=EDGE_CURVE('',#14677,#14678,#1803,.T.);
#18978=EDGE_CURVE('',#14679,#14678,#9553,.T.);
#18979=EDGE_CURVE('',#14680,#14679,#1804,.T.);
#18980=EDGE_CURVE('',#14681,#14680,#9554,.T.);
#18981=EDGE_CURVE('',#14681,#14682,#1805,.T.);
#18982=EDGE_CURVE('',#14683,#14682,#9555,.T.);
#18983=EDGE_CURVE('',#14684,#14683,#1806,.T.);
#18984=EDGE_CURVE('',#14685,#14684,#9556,.T.);
#18985=EDGE_CURVE('',#14685,#14686,#1807,.T.);
#18986=EDGE_CURVE('',#14687,#14686,#9557,.T.);
#18987=EDGE_CURVE('',#14688,#14687,#1808,.T.);
#18988=EDGE_CURVE('',#14689,#14688,#9558,.T.);
#18989=EDGE_CURVE('',#14689,#14690,#1809,.T.);
#18990=EDGE_CURVE('',#14691,#14690,#9559,.T.);
#18991=EDGE_CURVE('',#14692,#14691,#1810,.T.);
#18992=EDGE_CURVE('',#14693,#14692,#9560,.T.);
#18993=EDGE_CURVE('',#14693,#14694,#1811,.T.);
#18994=EDGE_CURVE('',#14695,#14694,#9561,.T.);
#18995=EDGE_CURVE('',#14696,#14695,#1812,.T.);
#18996=EDGE_CURVE('',#14697,#14696,#9562,.T.);
#18997=EDGE_CURVE('',#14697,#14698,#1813,.T.);
#18998=EDGE_CURVE('',#14699,#14698,#9563,.T.);
#18999=EDGE_CURVE('',#14700,#14699,#1814,.T.);
#19000=EDGE_CURVE('',#14701,#14700,#9564,.T.);
#19001=EDGE_CURVE('',#14701,#14702,#1815,.T.);
#19002=EDGE_CURVE('',#14643,#14702,#9565,.T.);
#19003=EDGE_CURVE('',#14642,#14635,#1816,.T.);
#19004=EDGE_CURVE('',#14702,#14703,#9566,.F.);
#19005=EDGE_CURVE('',#14703,#14644,#9567,.T.);
#19006=EDGE_CURVE('',#14704,#14703,#1817,.T.);
#19007=EDGE_CURVE('',#14705,#14704,#9568,.T.);
#19008=EDGE_CURVE('',#14706,#14705,#3223,.T.);
#19009=EDGE_CURVE('',#14645,#14706,#1818,.T.);
#19010=EDGE_CURVE('',#14700,#14705,#205,.T.);
#19011=EDGE_CURVE('',#14704,#14701,#9569,.F.);
#19012=EDGE_CURVE('',#14707,#14699,#206,.T.);
#19013=EDGE_CURVE('',#14707,#14708,#3224,.T.);
#19014=EDGE_CURVE('',#14706,#14708,#1819,.T.);
#19015=EDGE_CURVE('',#14698,#14709,#9570,.F.);
#19016=EDGE_CURVE('',#14709,#14707,#9571,.T.);
#19017=EDGE_CURVE('',#14710,#14709,#1820,.T.);
#19018=EDGE_CURVE('',#14711,#14710,#9572,.T.);
#19019=EDGE_CURVE('',#14712,#14711,#3225,.T.);
#19020=EDGE_CURVE('',#14708,#14712,#1821,.T.);
#19021=EDGE_CURVE('',#14696,#14711,#207,.T.);
#19022=EDGE_CURVE('',#14710,#14697,#9573,.F.);
#19023=EDGE_CURVE('',#14713,#14695,#208,.T.);
#19024=EDGE_CURVE('',#14713,#14714,#3226,.T.);
#19025=EDGE_CURVE('',#14712,#14714,#1822,.T.);
#19026=EDGE_CURVE('',#14694,#14715,#9574,.F.);
#19027=EDGE_CURVE('',#14715,#14713,#9575,.T.);
#19028=EDGE_CURVE('',#14716,#14715,#1823,.T.);
#19029=EDGE_CURVE('',#14717,#14716,#9576,.T.);
#19030=EDGE_CURVE('',#14718,#14717,#3227,.T.);
#19031=EDGE_CURVE('',#14714,#14718,#1824,.T.);
#19032=EDGE_CURVE('',#14692,#14717,#209,.T.);
#19033=EDGE_CURVE('',#14716,#14693,#9577,.F.);
#19034=EDGE_CURVE('',#14719,#14691,#210,.T.);
#19035=EDGE_CURVE('',#14719,#14720,#3228,.T.);
#19036=EDGE_CURVE('',#14718,#14720,#1825,.T.);
#19037=EDGE_CURVE('',#14690,#14721,#9578,.F.);
#19038=EDGE_CURVE('',#14721,#14719,#9579,.T.);
#19039=EDGE_CURVE('',#14722,#14721,#1826,.T.);
#19040=EDGE_CURVE('',#14723,#14722,#9580,.T.);
#19041=EDGE_CURVE('',#14724,#14723,#3229,.T.);
#19042=EDGE_CURVE('',#14720,#14724,#1827,.T.);
#19043=EDGE_CURVE('',#14688,#14723,#211,.T.);
#19044=EDGE_CURVE('',#14722,#14689,#9581,.F.);
#19045=EDGE_CURVE('',#14725,#14687,#212,.T.);
#19046=EDGE_CURVE('',#14725,#14726,#3230,.T.);
#19047=EDGE_CURVE('',#14724,#14726,#1828,.T.);
#19048=EDGE_CURVE('',#14686,#14727,#9582,.F.);
#19049=EDGE_CURVE('',#14727,#14725,#9583,.T.);
#19050=EDGE_CURVE('',#14728,#14727,#1829,.T.);
#19051=EDGE_CURVE('',#14729,#14728,#9584,.T.);
#19052=EDGE_CURVE('',#14730,#14729,#3231,.T.);
#19053=EDGE_CURVE('',#14726,#14730,#1830,.T.);
#19054=EDGE_CURVE('',#14684,#14729,#213,.T.);
#19055=EDGE_CURVE('',#14728,#14685,#9585,.F.);
#19056=EDGE_CURVE('',#14731,#14683,#214,.T.);
#19057=EDGE_CURVE('',#14731,#14732,#3232,.T.);
#19058=EDGE_CURVE('',#14730,#14732,#1831,.T.);
#19059=EDGE_CURVE('',#14682,#14733,#9586,.F.);
#19060=EDGE_CURVE('',#14733,#14731,#9587,.T.);
#19061=EDGE_CURVE('',#14734,#14733,#1832,.T.);
#19062=EDGE_CURVE('',#14735,#14734,#9588,.T.);
#19063=EDGE_CURVE('',#14736,#14735,#3233,.T.);
#19064=EDGE_CURVE('',#14732,#14736,#1833,.T.);
#19065=EDGE_CURVE('',#14680,#14735,#215,.T.);
#19066=EDGE_CURVE('',#14734,#14681,#9589,.F.);
#19067=EDGE_CURVE('',#14737,#14679,#216,.T.);
#19068=EDGE_CURVE('',#14737,#14738,#3234,.T.);
#19069=EDGE_CURVE('',#14736,#14738,#1834,.T.);
#19070=EDGE_CURVE('',#14678,#14739,#9590,.F.);
#19071=EDGE_CURVE('',#14739,#14737,#9591,.T.);
#19072=EDGE_CURVE('',#14740,#14739,#1835,.T.);
#19073=EDGE_CURVE('',#14741,#14740,#9592,.T.);
#19074=EDGE_CURVE('',#14742,#14741,#3235,.T.);
#19075=EDGE_CURVE('',#14738,#14742,#1836,.T.);
#19076=EDGE_CURVE('',#14676,#14741,#217,.T.);
#19077=EDGE_CURVE('',#14740,#14677,#9593,.F.);
#19078=EDGE_CURVE('',#14743,#14673,#218,.T.);
#19079=EDGE_CURVE('',#14743,#14744,#3236,.T.);
#19080=EDGE_CURVE('',#14742,#14744,#1837,.T.);
#19081=EDGE_CURVE('',#14672,#14745,#9594,.F.);
#19082=EDGE_CURVE('',#14745,#14743,#9595,.T.);
#19083=EDGE_CURVE('',#14746,#14745,#1838,.T.);
#19084=EDGE_CURVE('',#14747,#14746,#9596,.T.);
#19085=EDGE_CURVE('',#14748,#14747,#3237,.T.);
#19086=EDGE_CURVE('',#14744,#14748,#1839,.T.);
#19087=EDGE_CURVE('',#14670,#14747,#219,.T.);
#19088=EDGE_CURVE('',#14746,#14671,#9597,.F.);
#19089=EDGE_CURVE('',#14749,#14669,#220,.T.);
#19090=EDGE_CURVE('',#14749,#14750,#3238,.T.);
#19091=EDGE_CURVE('',#14748,#14750,#1840,.T.);
#19092=EDGE_CURVE('',#14668,#14751,#9598,.F.);
#19093=EDGE_CURVE('',#14751,#14749,#9599,.T.);
#19094=EDGE_CURVE('',#14752,#14751,#1841,.T.);
#19095=EDGE_CURVE('',#14753,#14752,#9600,.T.);
#19096=EDGE_CURVE('',#14754,#14753,#3239,.T.);
#19097=EDGE_CURVE('',#14750,#14754,#1842,.T.);
#19098=EDGE_CURVE('',#14666,#14753,#221,.T.);
#19099=EDGE_CURVE('',#14752,#14667,#9601,.F.);
#19100=EDGE_CURVE('',#14755,#14665,#222,.T.);
#19101=EDGE_CURVE('',#14755,#14756,#3240,.T.);
#19102=EDGE_CURVE('',#14754,#14756,#1843,.T.);
#19103=EDGE_CURVE('',#14664,#14757,#9602,.F.);
#19104=EDGE_CURVE('',#14757,#14755,#9603,.T.);
#19105=EDGE_CURVE('',#14758,#14757,#1844,.T.);
#19106=EDGE_CURVE('',#14759,#14758,#9604,.T.);
#19107=EDGE_CURVE('',#14760,#14759,#3241,.T.);
#19108=EDGE_CURVE('',#14756,#14760,#1845,.T.);
#19109=EDGE_CURVE('',#14662,#14759,#223,.T.);
#19110=EDGE_CURVE('',#14758,#14663,#9605,.F.);
#19111=EDGE_CURVE('',#14761,#14661,#224,.T.);
#19112=EDGE_CURVE('',#14761,#14762,#3242,.T.);
#19113=EDGE_CURVE('',#14760,#14762,#1846,.T.);
#19114=EDGE_CURVE('',#14660,#14763,#9606,.F.);
#19115=EDGE_CURVE('',#14763,#14761,#9607,.T.);
#19116=EDGE_CURVE('',#14764,#14763,#1847,.T.);
#19117=EDGE_CURVE('',#14765,#14764,#9608,.T.);
#19118=EDGE_CURVE('',#14766,#14765,#3243,.T.);
#19119=EDGE_CURVE('',#14762,#14766,#1848,.T.);
#19120=EDGE_CURVE('',#14658,#14765,#225,.T.);
#19121=EDGE_CURVE('',#14764,#14659,#9609,.F.);
#19122=EDGE_CURVE('',#14767,#14657,#226,.T.);
#19123=EDGE_CURVE('',#14767,#14768,#3244,.T.);
#19124=EDGE_CURVE('',#14766,#14768,#1849,.T.);
#19125=EDGE_CURVE('',#14656,#14769,#9610,.F.);
#19126=EDGE_CURVE('',#14769,#14767,#9611,.T.);
#19127=EDGE_CURVE('',#14770,#14769,#1850,.T.);
#19128=EDGE_CURVE('',#14771,#14770,#9612,.T.);
#19129=EDGE_CURVE('',#14772,#14771,#3245,.T.);
#19130=EDGE_CURVE('',#14768,#14772,#1851,.T.);
#19131=EDGE_CURVE('',#14654,#14771,#227,.T.);
#19132=EDGE_CURVE('',#14770,#14655,#9613,.F.);
#19133=EDGE_CURVE('',#14773,#14653,#228,.T.);
#19134=EDGE_CURVE('',#14773,#14774,#3246,.T.);
#19135=EDGE_CURVE('',#14772,#14774,#1852,.T.);
#19136=EDGE_CURVE('',#14652,#14775,#9614,.F.);
#19137=EDGE_CURVE('',#14775,#14773,#9615,.T.);
#19138=EDGE_CURVE('',#14776,#14775,#1853,.T.);
#19139=EDGE_CURVE('',#14777,#14776,#9616,.T.);
#19140=EDGE_CURVE('',#14778,#14777,#3247,.T.);
#19141=EDGE_CURVE('',#14774,#14778,#1854,.T.);
#19142=EDGE_CURVE('',#14650,#14777,#229,.T.);
#19143=EDGE_CURVE('',#14776,#14651,#9617,.F.);
#19144=EDGE_CURVE('',#14779,#14649,#230,.T.);
#19145=EDGE_CURVE('',#14779,#14780,#3248,.T.);
#19146=EDGE_CURVE('',#14778,#14780,#1855,.T.);
#19147=EDGE_CURVE('',#14648,#14781,#9618,.F.);
#19148=EDGE_CURVE('',#14781,#14779,#9619,.T.);
#19149=EDGE_CURVE('',#14782,#14781,#1856,.T.);
#19150=EDGE_CURVE('',#14783,#14782,#9620,.T.);
#19151=EDGE_CURVE('',#14784,#14783,#3249,.T.);
#19152=EDGE_CURVE('',#14780,#14784,#1857,.T.);
#19153=EDGE_CURVE('',#14646,#14783,#231,.T.);
#19154=EDGE_CURVE('',#14782,#14647,#9621,.F.);
#19155=EDGE_CURVE('',#14785,#14786,#9622,.T.);
#19156=EDGE_CURVE('',#14786,#14787,#9623,.T.);
#19157=EDGE_CURVE('',#14787,#14788,#9624,.T.);
#19158=EDGE_CURVE('',#14785,#14788,#9625,.T.);
#19159=EDGE_CURVE('',#14786,#14789,#9626,.T.);
#19160=EDGE_CURVE('',#14789,#14790,#9627,.T.);
#19161=EDGE_CURVE('',#14790,#14787,#9628,.T.);
#19162=EDGE_CURVE('',#14791,#14792,#9629,.T.);
#19163=EDGE_CURVE('',#14792,#14793,#9630,.T.);
#19164=EDGE_CURVE('',#14793,#14794,#9631,.T.);
#19165=EDGE_CURVE('',#14794,#14791,#9632,.T.);
#19166=EDGE_CURVE('',#14795,#14793,#9633,.T.);
#19167=EDGE_CURVE('',#14792,#14796,#9634,.T.);
#19168=EDGE_CURVE('',#14796,#14795,#9635,.T.);
#19169=EDGE_CURVE('',#14789,#14791,#9636,.T.);
#19170=EDGE_CURVE('',#14794,#14790,#9637,.T.);
#19171=EDGE_CURVE('',#14788,#14795,#9638,.T.);
#19172=EDGE_CURVE('',#14796,#14785,#9639,.T.);
#19173=EDGE_CURVE('',#14790,#14797,#9640,.T.);
#19174=EDGE_CURVE('',#14797,#14798,#9641,.T.);
#19175=EDGE_CURVE('',#14787,#14798,#9642,.T.);
#19176=EDGE_CURVE('',#14794,#14799,#9643,.T.);
#19177=EDGE_CURVE('',#14799,#14797,#9644,.T.);
#19178=EDGE_CURVE('',#14793,#14800,#9645,.T.);
#19179=EDGE_CURVE('',#14800,#14799,#9646,.T.);
#19180=EDGE_CURVE('',#14784,#14640,#1858,.T.);
#19181=EDGE_CURVE('',#14795,#14801,#9647,.T.);
#19182=EDGE_CURVE('',#14801,#14800,#9648,.T.);
#19183=EDGE_CURVE('',#14788,#14802,#9649,.T.);
#19184=EDGE_CURVE('',#14802,#14801,#9650,.T.);
#19185=EDGE_CURVE('',#14798,#14802,#9651,.T.);
#19186=EDGE_CURVE('',#14803,#14803,#1859,.T.);
#19187=EDGE_CURVE('',#14803,#14632,#9652,.T.);
#19188=EDGE_CURVE('',#14804,#14804,#1860,.T.);
#19189=EDGE_CURVE('',#14804,#14803,#9653,.T.);
#19190=EDGE_CURVE('',#14805,#14805,#1861,.T.);
#19191=EDGE_CURVE('',#14675,#14805,#9654,.T.);
#27399=ORIENTED_EDGE('',*,*,#18921,.T.);
#27400=ORIENTED_EDGE('',*,*,#18922,.T.);
#27401=ORIENTED_EDGE('',*,*,#18923,.T.);
#27402=ORIENTED_EDGE('',*,*,#18924,.T.);
#27403=ORIENTED_EDGE('',*,*,#18922,.F.);
#27404=ORIENTED_EDGE('',*,*,#18925,.T.);
#27405=ORIENTED_EDGE('',*,*,#18926,.T.);
#27406=ORIENTED_EDGE('',*,*,#18923,.F.);
#27407=ORIENTED_EDGE('',*,*,#18924,.F.);
#27408=ORIENTED_EDGE('',*,*,#18926,.F.);
#27409=ORIENTED_EDGE('',*,*,#18927,.F.);
#27410=ORIENTED_EDGE('',*,*,#18921,.F.);
#27411=ORIENTED_EDGE('',*,*,#18928,.T.);
#27412=ORIENTED_EDGE('',*,*,#18929,.T.);
#27413=ORIENTED_EDGE('',*,*,#18930,.T.);
#27414=ORIENTED_EDGE('',*,*,#18931,.T.);
#27415=ORIENTED_EDGE('',*,*,#18931,.F.);
#27416=ORIENTED_EDGE('',*,*,#18932,.F.);
#27417=ORIENTED_EDGE('',*,*,#18933,.F.);
#27418=ORIENTED_EDGE('',*,*,#18934,.F.);
#27419=ORIENTED_EDGE('',*,*,#18935,.F.);
#27420=ORIENTED_EDGE('',*,*,#18936,.F.);
#27421=ORIENTED_EDGE('',*,*,#18937,.T.);
#27422=ORIENTED_EDGE('',*,*,#18933,.T.);
#27423=ORIENTED_EDGE('',*,*,#18938,.T.);
#27424=ORIENTED_EDGE('',*,*,#18939,.T.);
#27425=ORIENTED_EDGE('',*,*,#18937,.F.);
#27426=ORIENTED_EDGE('',*,*,#18940,.T.);
#27427=ORIENTED_EDGE('',*,*,#18941,.F.);
#27428=ORIENTED_EDGE('',*,*,#18942,.T.);
#27429=ORIENTED_EDGE('',*,*,#18943,.F.);
#27430=ORIENTED_EDGE('',*,*,#18934,.T.);
#27431=ORIENTED_EDGE('',*,*,#18929,.F.);
#27432=ORIENTED_EDGE('',*,*,#18944,.F.);
#27433=ORIENTED_EDGE('',*,*,#18945,.F.);
#27434=ORIENTED_EDGE('',*,*,#18946,.T.);
#27435=ORIENTED_EDGE('',*,*,#18947,.F.);
#27436=ORIENTED_EDGE('',*,*,#18948,.F.);
#27437=ORIENTED_EDGE('',*,*,#18949,.F.);
#27438=ORIENTED_EDGE('',*,*,#18950,.T.);
#27439=ORIENTED_EDGE('',*,*,#18951,.F.);
#27440=ORIENTED_EDGE('',*,*,#18952,.F.);
#27441=ORIENTED_EDGE('',*,*,#18953,.F.);
#27442=ORIENTED_EDGE('',*,*,#18954,.T.);
#27443=ORIENTED_EDGE('',*,*,#18955,.F.);
#27444=ORIENTED_EDGE('',*,*,#18956,.F.);
#27445=ORIENTED_EDGE('',*,*,#18957,.F.);
#27446=ORIENTED_EDGE('',*,*,#18958,.T.);
#27447=ORIENTED_EDGE('',*,*,#18959,.F.);
#27448=ORIENTED_EDGE('',*,*,#18960,.F.);
#27449=ORIENTED_EDGE('',*,*,#18961,.F.);
#27450=ORIENTED_EDGE('',*,*,#18962,.T.);
#27451=ORIENTED_EDGE('',*,*,#18963,.F.);
#27452=ORIENTED_EDGE('',*,*,#18964,.F.);
#27453=ORIENTED_EDGE('',*,*,#18965,.F.);
#27454=ORIENTED_EDGE('',*,*,#18966,.T.);
#27455=ORIENTED_EDGE('',*,*,#18967,.F.);
#27456=ORIENTED_EDGE('',*,*,#18968,.F.);
#27457=ORIENTED_EDGE('',*,*,#18969,.F.);
#27458=ORIENTED_EDGE('',*,*,#18970,.T.);
#27459=ORIENTED_EDGE('',*,*,#18971,.F.);
#27460=ORIENTED_EDGE('',*,*,#18972,.F.);
#27461=ORIENTED_EDGE('',*,*,#18973,.T.);
#27462=ORIENTED_EDGE('',*,*,#18974,.T.);
#27463=ORIENTED_EDGE('',*,*,#18973,.F.);
#27464=ORIENTED_EDGE('',*,*,#18975,.F.);
#27465=ORIENTED_EDGE('',*,*,#18976,.F.);
#27466=ORIENTED_EDGE('',*,*,#18977,.T.);
#27467=ORIENTED_EDGE('',*,*,#18978,.F.);
#27468=ORIENTED_EDGE('',*,*,#18979,.F.);
#27469=ORIENTED_EDGE('',*,*,#18980,.F.);
#27470=ORIENTED_EDGE('',*,*,#18981,.T.);
#27471=ORIENTED_EDGE('',*,*,#18982,.F.);
#27472=ORIENTED_EDGE('',*,*,#18983,.F.);
#27473=ORIENTED_EDGE('',*,*,#18984,.F.);
#27474=ORIENTED_EDGE('',*,*,#18985,.T.);
#27475=ORIENTED_EDGE('',*,*,#18986,.F.);
#27476=ORIENTED_EDGE('',*,*,#18987,.F.);
#27477=ORIENTED_EDGE('',*,*,#18988,.F.);
#27478=ORIENTED_EDGE('',*,*,#18989,.T.);
#27479=ORIENTED_EDGE('',*,*,#18990,.F.);
#27480=ORIENTED_EDGE('',*,*,#18991,.F.);
#27481=ORIENTED_EDGE('',*,*,#18992,.F.);
#27482=ORIENTED_EDGE('',*,*,#18993,.T.);
#27483=ORIENTED_EDGE('',*,*,#18994,.F.);
#27484=ORIENTED_EDGE('',*,*,#18995,.F.);
#27485=ORIENTED_EDGE('',*,*,#18996,.F.);
#27486=ORIENTED_EDGE('',*,*,#18997,.T.);
#27487=ORIENTED_EDGE('',*,*,#18998,.F.);
#27488=ORIENTED_EDGE('',*,*,#18999,.F.);
#27489=ORIENTED_EDGE('',*,*,#19000,.F.);
#27490=ORIENTED_EDGE('',*,*,#19001,.T.);
#27491=ORIENTED_EDGE('',*,*,#19002,.F.);
#27492=ORIENTED_EDGE('',*,*,#18940,.F.);
#27493=ORIENTED_EDGE('',*,*,#18939,.F.);
#27494=ORIENTED_EDGE('',*,*,#19003,.T.);
#27495=ORIENTED_EDGE('',*,*,#18941,.T.);
#27496=ORIENTED_EDGE('',*,*,#19002,.T.);
#27497=ORIENTED_EDGE('',*,*,#19004,.T.);
#27498=ORIENTED_EDGE('',*,*,#19005,.T.);
#27499=ORIENTED_EDGE('',*,*,#19005,.F.);
#27500=ORIENTED_EDGE('',*,*,#19006,.F.);
#27501=ORIENTED_EDGE('',*,*,#19007,.F.);
#27502=ORIENTED_EDGE('',*,*,#19008,.F.);
#27503=ORIENTED_EDGE('',*,*,#19009,.F.);
#27504=ORIENTED_EDGE('',*,*,#18942,.F.);
#27505=ORIENTED_EDGE('',*,*,#19010,.T.);
#27506=ORIENTED_EDGE('',*,*,#19007,.T.);
#27507=ORIENTED_EDGE('',*,*,#19011,.T.);
#27508=ORIENTED_EDGE('',*,*,#19000,.T.);
#27509=ORIENTED_EDGE('',*,*,#19010,.F.);
#27510=ORIENTED_EDGE('',*,*,#18999,.T.);
#27511=ORIENTED_EDGE('',*,*,#19012,.F.);
#27512=ORIENTED_EDGE('',*,*,#19013,.T.);
#27513=ORIENTED_EDGE('',*,*,#19014,.F.);
#27514=ORIENTED_EDGE('',*,*,#19008,.T.);
#27515=ORIENTED_EDGE('',*,*,#19012,.T.);
#27516=ORIENTED_EDGE('',*,*,#18998,.T.);
#27517=ORIENTED_EDGE('',*,*,#19015,.T.);
#27518=ORIENTED_EDGE('',*,*,#19016,.T.);
#27519=ORIENTED_EDGE('',*,*,#19016,.F.);
#27520=ORIENTED_EDGE('',*,*,#19017,.F.);
#27521=ORIENTED_EDGE('',*,*,#19018,.F.);
#27522=ORIENTED_EDGE('',*,*,#19019,.F.);
#27523=ORIENTED_EDGE('',*,*,#19020,.F.);
#27524=ORIENTED_EDGE('',*,*,#19013,.F.);
#27525=ORIENTED_EDGE('',*,*,#19021,.T.);
#27526=ORIENTED_EDGE('',*,*,#19018,.T.);
#27527=ORIENTED_EDGE('',*,*,#19022,.T.);
#27528=ORIENTED_EDGE('',*,*,#18996,.T.);
#27529=ORIENTED_EDGE('',*,*,#19021,.F.);
#27530=ORIENTED_EDGE('',*,*,#18995,.T.);
#27531=ORIENTED_EDGE('',*,*,#19023,.F.);
#27532=ORIENTED_EDGE('',*,*,#19024,.T.);
#27533=ORIENTED_EDGE('',*,*,#19025,.F.);
#27534=ORIENTED_EDGE('',*,*,#19019,.T.);
#27535=ORIENTED_EDGE('',*,*,#19023,.T.);
#27536=ORIENTED_EDGE('',*,*,#18994,.T.);
#27537=ORIENTED_EDGE('',*,*,#19026,.T.);
#27538=ORIENTED_EDGE('',*,*,#19027,.T.);
#27539=ORIENTED_EDGE('',*,*,#19027,.F.);
#27540=ORIENTED_EDGE('',*,*,#19028,.F.);
#27541=ORIENTED_EDGE('',*,*,#19029,.F.);
#27542=ORIENTED_EDGE('',*,*,#19030,.F.);
#27543=ORIENTED_EDGE('',*,*,#19031,.F.);
#27544=ORIENTED_EDGE('',*,*,#19024,.F.);
#27545=ORIENTED_EDGE('',*,*,#19032,.T.);
#27546=ORIENTED_EDGE('',*,*,#19029,.T.);
#27547=ORIENTED_EDGE('',*,*,#19033,.T.);
#27548=ORIENTED_EDGE('',*,*,#18992,.T.);
#27549=ORIENTED_EDGE('',*,*,#19032,.F.);
#27550=ORIENTED_EDGE('',*,*,#18991,.T.);
#27551=ORIENTED_EDGE('',*,*,#19034,.F.);
#27552=ORIENTED_EDGE('',*,*,#19035,.T.);
#27553=ORIENTED_EDGE('',*,*,#19036,.F.);
#27554=ORIENTED_EDGE('',*,*,#19030,.T.);
#27555=ORIENTED_EDGE('',*,*,#19034,.T.);
#27556=ORIENTED_EDGE('',*,*,#18990,.T.);
#27557=ORIENTED_EDGE('',*,*,#19037,.T.);
#27558=ORIENTED_EDGE('',*,*,#19038,.T.);
#27559=ORIENTED_EDGE('',*,*,#19038,.F.);
#27560=ORIENTED_EDGE('',*,*,#19039,.F.);
#27561=ORIENTED_EDGE('',*,*,#19040,.F.);
#27562=ORIENTED_EDGE('',*,*,#19041,.F.);
#27563=ORIENTED_EDGE('',*,*,#19042,.F.);
#27564=ORIENTED_EDGE('',*,*,#19035,.F.);
#27565=ORIENTED_EDGE('',*,*,#19043,.T.);
#27566=ORIENTED_EDGE('',*,*,#19040,.T.);
#27567=ORIENTED_EDGE('',*,*,#19044,.T.);
#27568=ORIENTED_EDGE('',*,*,#18988,.T.);
#27569=ORIENTED_EDGE('',*,*,#19043,.F.);
#27570=ORIENTED_EDGE('',*,*,#18987,.T.);
#27571=ORIENTED_EDGE('',*,*,#19045,.F.);
#27572=ORIENTED_EDGE('',*,*,#19046,.T.);
#27573=ORIENTED_EDGE('',*,*,#19047,.F.);
#27574=ORIENTED_EDGE('',*,*,#19041,.T.);
#27575=ORIENTED_EDGE('',*,*,#19045,.T.);
#27576=ORIENTED_EDGE('',*,*,#18986,.T.);
#27577=ORIENTED_EDGE('',*,*,#19048,.T.);
#27578=ORIENTED_EDGE('',*,*,#19049,.T.);
#27579=ORIENTED_EDGE('',*,*,#19049,.F.);
#27580=ORIENTED_EDGE('',*,*,#19050,.F.);
#27581=ORIENTED_EDGE('',*,*,#19051,.F.);
#27582=ORIENTED_EDGE('',*,*,#19052,.F.);
#27583=ORIENTED_EDGE('',*,*,#19053,.F.);
#27584=ORIENTED_EDGE('',*,*,#19046,.F.);
#27585=ORIENTED_EDGE('',*,*,#19054,.T.);
#27586=ORIENTED_EDGE('',*,*,#19051,.T.);
#27587=ORIENTED_EDGE('',*,*,#19055,.T.);
#27588=ORIENTED_EDGE('',*,*,#18984,.T.);
#27589=ORIENTED_EDGE('',*,*,#19054,.F.);
#27590=ORIENTED_EDGE('',*,*,#18983,.T.);
#27591=ORIENTED_EDGE('',*,*,#19056,.F.);
#27592=ORIENTED_EDGE('',*,*,#19057,.T.);
#27593=ORIENTED_EDGE('',*,*,#19058,.F.);
#27594=ORIENTED_EDGE('',*,*,#19052,.T.);
#27595=ORIENTED_EDGE('',*,*,#19056,.T.);
#27596=ORIENTED_EDGE('',*,*,#18982,.T.);
#27597=ORIENTED_EDGE('',*,*,#19059,.T.);
#27598=ORIENTED_EDGE('',*,*,#19060,.T.);
#27599=ORIENTED_EDGE('',*,*,#19060,.F.);
#27600=ORIENTED_EDGE('',*,*,#19061,.F.);
#27601=ORIENTED_EDGE('',*,*,#19062,.F.);
#27602=ORIENTED_EDGE('',*,*,#19063,.F.);
#27603=ORIENTED_EDGE('',*,*,#19064,.F.);
#27604=ORIENTED_EDGE('',*,*,#19057,.F.);
#27605=ORIENTED_EDGE('',*,*,#19065,.T.);
#27606=ORIENTED_EDGE('',*,*,#19062,.T.);
#27607=ORIENTED_EDGE('',*,*,#19066,.T.);
#27608=ORIENTED_EDGE('',*,*,#18980,.T.);
#27609=ORIENTED_EDGE('',*,*,#19065,.F.);
#27610=ORIENTED_EDGE('',*,*,#18979,.T.);
#27611=ORIENTED_EDGE('',*,*,#19067,.F.);
#27612=ORIENTED_EDGE('',*,*,#19068,.T.);
#27613=ORIENTED_EDGE('',*,*,#19069,.F.);
#27614=ORIENTED_EDGE('',*,*,#19063,.T.);
#27615=ORIENTED_EDGE('',*,*,#19067,.T.);
#27616=ORIENTED_EDGE('',*,*,#18978,.T.);
#27617=ORIENTED_EDGE('',*,*,#19070,.T.);
#27618=ORIENTED_EDGE('',*,*,#19071,.T.);
#27619=ORIENTED_EDGE('',*,*,#19071,.F.);
#27620=ORIENTED_EDGE('',*,*,#19072,.F.);
#27621=ORIENTED_EDGE('',*,*,#19073,.F.);
#27622=ORIENTED_EDGE('',*,*,#19074,.F.);
#27623=ORIENTED_EDGE('',*,*,#19075,.F.);
#27624=ORIENTED_EDGE('',*,*,#19068,.F.);
#27625=ORIENTED_EDGE('',*,*,#19076,.T.);
#27626=ORIENTED_EDGE('',*,*,#19073,.T.);
#27627=ORIENTED_EDGE('',*,*,#19077,.T.);
#27628=ORIENTED_EDGE('',*,*,#18976,.T.);
#27629=ORIENTED_EDGE('',*,*,#19076,.F.);
#27630=ORIENTED_EDGE('',*,*,#18975,.T.);
#27631=ORIENTED_EDGE('',*,*,#18972,.T.);
#27632=ORIENTED_EDGE('',*,*,#19078,.F.);
#27633=ORIENTED_EDGE('',*,*,#19079,.T.);
#27634=ORIENTED_EDGE('',*,*,#19080,.F.);
#27635=ORIENTED_EDGE('',*,*,#19074,.T.);
#27636=ORIENTED_EDGE('',*,*,#19078,.T.);
#27637=ORIENTED_EDGE('',*,*,#18971,.T.);
#27638=ORIENTED_EDGE('',*,*,#19081,.T.);
#27639=ORIENTED_EDGE('',*,*,#19082,.T.);
#27640=ORIENTED_EDGE('',*,*,#19082,.F.);
#27641=ORIENTED_EDGE('',*,*,#19083,.F.);
#27642=ORIENTED_EDGE('',*,*,#19084,.F.);
#27643=ORIENTED_EDGE('',*,*,#19085,.F.);
#27644=ORIENTED_EDGE('',*,*,#19086,.F.);
#27645=ORIENTED_EDGE('',*,*,#19079,.F.);
#27646=ORIENTED_EDGE('',*,*,#19087,.T.);
#27647=ORIENTED_EDGE('',*,*,#19084,.T.);
#27648=ORIENTED_EDGE('',*,*,#19088,.T.);
#27649=ORIENTED_EDGE('',*,*,#18969,.T.);
#27650=ORIENTED_EDGE('',*,*,#19087,.F.);
#27651=ORIENTED_EDGE('',*,*,#18968,.T.);
#27652=ORIENTED_EDGE('',*,*,#19089,.F.);
#27653=ORIENTED_EDGE('',*,*,#19090,.T.);
#27654=ORIENTED_EDGE('',*,*,#19091,.F.);
#27655=ORIENTED_EDGE('',*,*,#19085,.T.);
#27656=ORIENTED_EDGE('',*,*,#19089,.T.);
#27657=ORIENTED_EDGE('',*,*,#18967,.T.);
#27658=ORIENTED_EDGE('',*,*,#19092,.T.);
#27659=ORIENTED_EDGE('',*,*,#19093,.T.);
#27660=ORIENTED_EDGE('',*,*,#19093,.F.);
#27661=ORIENTED_EDGE('',*,*,#19094,.F.);
#27662=ORIENTED_EDGE('',*,*,#19095,.F.);
#27663=ORIENTED_EDGE('',*,*,#19096,.F.);
#27664=ORIENTED_EDGE('',*,*,#19097,.F.);
#27665=ORIENTED_EDGE('',*,*,#19090,.F.);
#27666=ORIENTED_EDGE('',*,*,#19098,.T.);
#27667=ORIENTED_EDGE('',*,*,#19095,.T.);
#27668=ORIENTED_EDGE('',*,*,#19099,.T.);
#27669=ORIENTED_EDGE('',*,*,#18965,.T.);
#27670=ORIENTED_EDGE('',*,*,#19098,.F.);
#27671=ORIENTED_EDGE('',*,*,#18964,.T.);
#27672=ORIENTED_EDGE('',*,*,#19100,.F.);
#27673=ORIENTED_EDGE('',*,*,#19101,.T.);
#27674=ORIENTED_EDGE('',*,*,#19102,.F.);
#27675=ORIENTED_EDGE('',*,*,#19096,.T.);
#27676=ORIENTED_EDGE('',*,*,#19100,.T.);
#27677=ORIENTED_EDGE('',*,*,#18963,.T.);
#27678=ORIENTED_EDGE('',*,*,#19103,.T.);
#27679=ORIENTED_EDGE('',*,*,#19104,.T.);
#27680=ORIENTED_EDGE('',*,*,#19104,.F.);
#27681=ORIENTED_EDGE('',*,*,#19105,.F.);
#27682=ORIENTED_EDGE('',*,*,#19106,.F.);
#27683=ORIENTED_EDGE('',*,*,#19107,.F.);
#27684=ORIENTED_EDGE('',*,*,#19108,.F.);
#27685=ORIENTED_EDGE('',*,*,#19101,.F.);
#27686=ORIENTED_EDGE('',*,*,#19109,.T.);
#27687=ORIENTED_EDGE('',*,*,#19106,.T.);
#27688=ORIENTED_EDGE('',*,*,#19110,.T.);
#27689=ORIENTED_EDGE('',*,*,#18961,.T.);
#27690=ORIENTED_EDGE('',*,*,#19109,.F.);
#27691=ORIENTED_EDGE('',*,*,#18960,.T.);
#27692=ORIENTED_EDGE('',*,*,#19111,.F.);
#27693=ORIENTED_EDGE('',*,*,#19112,.T.);
#27694=ORIENTED_EDGE('',*,*,#19113,.F.);
#27695=ORIENTED_EDGE('',*,*,#19107,.T.);
#27696=ORIENTED_EDGE('',*,*,#19111,.T.);
#27697=ORIENTED_EDGE('',*,*,#18959,.T.);
#27698=ORIENTED_EDGE('',*,*,#19114,.T.);
#27699=ORIENTED_EDGE('',*,*,#19115,.T.);
#27700=ORIENTED_EDGE('',*,*,#19115,.F.);
#27701=ORIENTED_EDGE('',*,*,#19116,.F.);
#27702=ORIENTED_EDGE('',*,*,#19117,.F.);
#27703=ORIENTED_EDGE('',*,*,#19118,.F.);
#27704=ORIENTED_EDGE('',*,*,#19119,.F.);
#27705=ORIENTED_EDGE('',*,*,#19112,.F.);
#27706=ORIENTED_EDGE('',*,*,#19120,.T.);
#27707=ORIENTED_EDGE('',*,*,#19117,.T.);
#27708=ORIENTED_EDGE('',*,*,#19121,.T.);
#27709=ORIENTED_EDGE('',*,*,#18957,.T.);
#27710=ORIENTED_EDGE('',*,*,#19120,.F.);
#27711=ORIENTED_EDGE('',*,*,#18956,.T.);
#27712=ORIENTED_EDGE('',*,*,#19122,.F.);
#27713=ORIENTED_EDGE('',*,*,#19123,.T.);
#27714=ORIENTED_EDGE('',*,*,#19124,.F.);
#27715=ORIENTED_EDGE('',*,*,#19118,.T.);
#27716=ORIENTED_EDGE('',*,*,#19122,.T.);
#27717=ORIENTED_EDGE('',*,*,#18955,.T.);
#27718=ORIENTED_EDGE('',*,*,#19125,.T.);
#27719=ORIENTED_EDGE('',*,*,#19126,.T.);
#27720=ORIENTED_EDGE('',*,*,#19126,.F.);
#27721=ORIENTED_EDGE('',*,*,#19127,.F.);
#27722=ORIENTED_EDGE('',*,*,#19128,.F.);
#27723=ORIENTED_EDGE('',*,*,#19129,.F.);
#27724=ORIENTED_EDGE('',*,*,#19130,.F.);
#27725=ORIENTED_EDGE('',*,*,#19123,.F.);
#27726=ORIENTED_EDGE('',*,*,#19131,.T.);
#27727=ORIENTED_EDGE('',*,*,#19128,.T.);
#27728=ORIENTED_EDGE('',*,*,#19132,.T.);
#27729=ORIENTED_EDGE('',*,*,#18953,.T.);
#27730=ORIENTED_EDGE('',*,*,#19131,.F.);
#27731=ORIENTED_EDGE('',*,*,#18952,.T.);
#27732=ORIENTED_EDGE('',*,*,#19133,.F.);
#27733=ORIENTED_EDGE('',*,*,#19134,.T.);
#27734=ORIENTED_EDGE('',*,*,#19135,.F.);
#27735=ORIENTED_EDGE('',*,*,#19129,.T.);
#27736=ORIENTED_EDGE('',*,*,#19133,.T.);
#27737=ORIENTED_EDGE('',*,*,#18951,.T.);
#27738=ORIENTED_EDGE('',*,*,#19136,.T.);
#27739=ORIENTED_EDGE('',*,*,#19137,.T.);
#27740=ORIENTED_EDGE('',*,*,#19137,.F.);
#27741=ORIENTED_EDGE('',*,*,#19138,.F.);
#27742=ORIENTED_EDGE('',*,*,#19139,.F.);
#27743=ORIENTED_EDGE('',*,*,#19140,.F.);
#27744=ORIENTED_EDGE('',*,*,#19141,.F.);
#27745=ORIENTED_EDGE('',*,*,#19134,.F.);
#27746=ORIENTED_EDGE('',*,*,#19142,.T.);
#27747=ORIENTED_EDGE('',*,*,#19139,.T.);
#27748=ORIENTED_EDGE('',*,*,#19143,.T.);
#27749=ORIENTED_EDGE('',*,*,#18949,.T.);
#27750=ORIENTED_EDGE('',*,*,#19142,.F.);
#27751=ORIENTED_EDGE('',*,*,#18948,.T.);
#27752=ORIENTED_EDGE('',*,*,#19144,.F.);
#27753=ORIENTED_EDGE('',*,*,#19145,.T.);
#27754=ORIENTED_EDGE('',*,*,#19146,.F.);
#27755=ORIENTED_EDGE('',*,*,#19140,.T.);
#27756=ORIENTED_EDGE('',*,*,#19144,.T.);
#27757=ORIENTED_EDGE('',*,*,#18947,.T.);
#27758=ORIENTED_EDGE('',*,*,#19147,.T.);
#27759=ORIENTED_EDGE('',*,*,#19148,.T.);
#27760=ORIENTED_EDGE('',*,*,#19148,.F.);
#27761=ORIENTED_EDGE('',*,*,#19149,.F.);
#27762=ORIENTED_EDGE('',*,*,#19150,.F.);
#27763=ORIENTED_EDGE('',*,*,#19151,.F.);
#27764=ORIENTED_EDGE('',*,*,#19152,.F.);
#27765=ORIENTED_EDGE('',*,*,#19145,.F.);
#27766=ORIENTED_EDGE('',*,*,#19153,.T.);
#27767=ORIENTED_EDGE('',*,*,#19150,.T.);
#27768=ORIENTED_EDGE('',*,*,#19154,.T.);
#27769=ORIENTED_EDGE('',*,*,#18945,.T.);
#27770=ORIENTED_EDGE('',*,*,#19155,.T.);
#27771=ORIENTED_EDGE('',*,*,#19156,.T.);
#27772=ORIENTED_EDGE('',*,*,#19157,.T.);
#27773=ORIENTED_EDGE('',*,*,#19158,.F.);
#27774=ORIENTED_EDGE('',*,*,#19159,.T.);
#27775=ORIENTED_EDGE('',*,*,#19160,.T.);
#27776=ORIENTED_EDGE('',*,*,#19161,.T.);
#27777=ORIENTED_EDGE('',*,*,#19156,.F.);
#27778=ORIENTED_EDGE('',*,*,#19162,.T.);
#27779=ORIENTED_EDGE('',*,*,#19163,.T.);
#27780=ORIENTED_EDGE('',*,*,#19164,.T.);
#27781=ORIENTED_EDGE('',*,*,#19165,.T.);
#27782=ORIENTED_EDGE('',*,*,#19166,.T.);
#27783=ORIENTED_EDGE('',*,*,#19163,.F.);
#27784=ORIENTED_EDGE('',*,*,#19167,.T.);
#27785=ORIENTED_EDGE('',*,*,#19168,.T.);
#27786=ORIENTED_EDGE('',*,*,#19169,.T.);
#27787=ORIENTED_EDGE('',*,*,#19165,.F.);
#27788=ORIENTED_EDGE('',*,*,#19170,.T.);
#27789=ORIENTED_EDGE('',*,*,#19160,.F.);
#27790=ORIENTED_EDGE('',*,*,#19171,.T.);
#27791=ORIENTED_EDGE('',*,*,#19168,.F.);
#27792=ORIENTED_EDGE('',*,*,#19172,.T.);
#27793=ORIENTED_EDGE('',*,*,#19158,.T.);
#27794=ORIENTED_EDGE('',*,*,#19161,.F.);
#27795=ORIENTED_EDGE('',*,*,#19173,.T.);
#27796=ORIENTED_EDGE('',*,*,#19174,.T.);
#27797=ORIENTED_EDGE('',*,*,#19175,.F.);
#27798=ORIENTED_EDGE('',*,*,#19170,.F.);
#27799=ORIENTED_EDGE('',*,*,#19176,.T.);
#27800=ORIENTED_EDGE('',*,*,#19177,.T.);
#27801=ORIENTED_EDGE('',*,*,#19173,.F.);
#27802=ORIENTED_EDGE('',*,*,#19164,.F.);
#27803=ORIENTED_EDGE('',*,*,#19178,.T.);
#27804=ORIENTED_EDGE('',*,*,#19179,.T.);
#27805=ORIENTED_EDGE('',*,*,#19176,.F.);
#27806=ORIENTED_EDGE('',*,*,#19152,.T.);
#27807=ORIENTED_EDGE('',*,*,#19180,.T.);
#27808=ORIENTED_EDGE('',*,*,#18935,.T.);
#27809=ORIENTED_EDGE('',*,*,#18943,.T.);
#27810=ORIENTED_EDGE('',*,*,#19009,.T.);
#27811=ORIENTED_EDGE('',*,*,#19014,.T.);
#27812=ORIENTED_EDGE('',*,*,#19020,.T.);
#27813=ORIENTED_EDGE('',*,*,#19025,.T.);
#27814=ORIENTED_EDGE('',*,*,#19031,.T.);
#27815=ORIENTED_EDGE('',*,*,#19036,.T.);
#27816=ORIENTED_EDGE('',*,*,#19042,.T.);
#27817=ORIENTED_EDGE('',*,*,#19047,.T.);
#27818=ORIENTED_EDGE('',*,*,#19053,.T.);
#27819=ORIENTED_EDGE('',*,*,#19058,.T.);
#27820=ORIENTED_EDGE('',*,*,#19064,.T.);
#27821=ORIENTED_EDGE('',*,*,#19069,.T.);
#27822=ORIENTED_EDGE('',*,*,#19075,.T.);
#27823=ORIENTED_EDGE('',*,*,#19080,.T.);
#27824=ORIENTED_EDGE('',*,*,#19086,.T.);
#27825=ORIENTED_EDGE('',*,*,#19091,.T.);
#27826=ORIENTED_EDGE('',*,*,#19097,.T.);
#27827=ORIENTED_EDGE('',*,*,#19102,.T.);
#27828=ORIENTED_EDGE('',*,*,#19108,.T.);
#27829=ORIENTED_EDGE('',*,*,#19113,.T.);
#27830=ORIENTED_EDGE('',*,*,#19119,.T.);
#27831=ORIENTED_EDGE('',*,*,#19124,.T.);
#27832=ORIENTED_EDGE('',*,*,#19130,.T.);
#27833=ORIENTED_EDGE('',*,*,#19135,.T.);
#27834=ORIENTED_EDGE('',*,*,#19141,.T.);
#27835=ORIENTED_EDGE('',*,*,#19146,.T.);
#27836=ORIENTED_EDGE('',*,*,#19162,.F.);
#27837=ORIENTED_EDGE('',*,*,#19169,.F.);
#27838=ORIENTED_EDGE('',*,*,#19159,.F.);
#27839=ORIENTED_EDGE('',*,*,#19155,.F.);
#27840=ORIENTED_EDGE('',*,*,#19172,.F.);
#27841=ORIENTED_EDGE('',*,*,#19167,.F.);
#27842=ORIENTED_EDGE('',*,*,#19166,.F.);
#27843=ORIENTED_EDGE('',*,*,#19181,.T.);
#27844=ORIENTED_EDGE('',*,*,#19182,.T.);
#27845=ORIENTED_EDGE('',*,*,#19178,.F.);
#27846=ORIENTED_EDGE('',*,*,#19171,.F.);
#27847=ORIENTED_EDGE('',*,*,#19183,.T.);
#27848=ORIENTED_EDGE('',*,*,#19184,.T.);
#27849=ORIENTED_EDGE('',*,*,#19181,.F.);
#27850=ORIENTED_EDGE('',*,*,#19157,.F.);
#27851=ORIENTED_EDGE('',*,*,#19175,.T.);
#27852=ORIENTED_EDGE('',*,*,#19185,.T.);
#27853=ORIENTED_EDGE('',*,*,#19183,.F.);
#27854=ORIENTED_EDGE('',*,*,#19177,.F.);
#27855=ORIENTED_EDGE('',*,*,#19179,.F.);
#27856=ORIENTED_EDGE('',*,*,#19182,.F.);
#27857=ORIENTED_EDGE('',*,*,#19184,.F.);
#27858=ORIENTED_EDGE('',*,*,#19185,.F.);
#27859=ORIENTED_EDGE('',*,*,#19174,.F.);
#27860=ORIENTED_EDGE('',*,*,#18946,.F.);
#27861=ORIENTED_EDGE('',*,*,#19154,.F.);
#27862=ORIENTED_EDGE('',*,*,#19149,.T.);
#27863=ORIENTED_EDGE('',*,*,#19147,.F.);
#27864=ORIENTED_EDGE('',*,*,#18950,.F.);
#27865=ORIENTED_EDGE('',*,*,#19143,.F.);
#27866=ORIENTED_EDGE('',*,*,#19138,.T.);
#27867=ORIENTED_EDGE('',*,*,#19136,.F.);
#27868=ORIENTED_EDGE('',*,*,#18954,.F.);
#27869=ORIENTED_EDGE('',*,*,#19132,.F.);
#27870=ORIENTED_EDGE('',*,*,#19127,.T.);
#27871=ORIENTED_EDGE('',*,*,#19125,.F.);
#27872=ORIENTED_EDGE('',*,*,#18958,.F.);
#27873=ORIENTED_EDGE('',*,*,#19121,.F.);
#27874=ORIENTED_EDGE('',*,*,#19116,.T.);
#27875=ORIENTED_EDGE('',*,*,#19114,.F.);
#27876=ORIENTED_EDGE('',*,*,#18962,.F.);
#27877=ORIENTED_EDGE('',*,*,#19110,.F.);
#27878=ORIENTED_EDGE('',*,*,#19105,.T.);
#27879=ORIENTED_EDGE('',*,*,#19103,.F.);
#27880=ORIENTED_EDGE('',*,*,#18966,.F.);
#27881=ORIENTED_EDGE('',*,*,#19099,.F.);
#27882=ORIENTED_EDGE('',*,*,#19094,.T.);
#27883=ORIENTED_EDGE('',*,*,#19092,.F.);
#27884=ORIENTED_EDGE('',*,*,#18970,.F.);
#27885=ORIENTED_EDGE('',*,*,#19088,.F.);
#27886=ORIENTED_EDGE('',*,*,#19083,.T.);
#27887=ORIENTED_EDGE('',*,*,#19081,.F.);
#27888=ORIENTED_EDGE('',*,*,#18977,.F.);
#27889=ORIENTED_EDGE('',*,*,#19077,.F.);
#27890=ORIENTED_EDGE('',*,*,#19072,.T.);
#27891=ORIENTED_EDGE('',*,*,#19070,.F.);
#27892=ORIENTED_EDGE('',*,*,#18981,.F.);
#27893=ORIENTED_EDGE('',*,*,#19066,.F.);
#27894=ORIENTED_EDGE('',*,*,#19061,.T.);
#27895=ORIENTED_EDGE('',*,*,#19059,.F.);
#27896=ORIENTED_EDGE('',*,*,#18985,.F.);
#27897=ORIENTED_EDGE('',*,*,#19055,.F.);
#27898=ORIENTED_EDGE('',*,*,#19050,.T.);
#27899=ORIENTED_EDGE('',*,*,#19048,.F.);
#27900=ORIENTED_EDGE('',*,*,#18989,.F.);
#27901=ORIENTED_EDGE('',*,*,#19044,.F.);
#27902=ORIENTED_EDGE('',*,*,#19039,.T.);
#27903=ORIENTED_EDGE('',*,*,#19037,.F.);
#27904=ORIENTED_EDGE('',*,*,#18993,.F.);
#27905=ORIENTED_EDGE('',*,*,#19033,.F.);
#27906=ORIENTED_EDGE('',*,*,#19028,.T.);
#27907=ORIENTED_EDGE('',*,*,#19026,.F.);
#27908=ORIENTED_EDGE('',*,*,#18997,.F.);
#27909=ORIENTED_EDGE('',*,*,#19022,.F.);
#27910=ORIENTED_EDGE('',*,*,#19017,.T.);
#27911=ORIENTED_EDGE('',*,*,#19015,.F.);
#27912=ORIENTED_EDGE('',*,*,#19001,.F.);
#27913=ORIENTED_EDGE('',*,*,#19011,.F.);
#27914=ORIENTED_EDGE('',*,*,#19006,.T.);
#27915=ORIENTED_EDGE('',*,*,#19004,.F.);
#27916=ORIENTED_EDGE('',*,*,#19003,.F.);
#27917=ORIENTED_EDGE('',*,*,#18938,.F.);
#27918=ORIENTED_EDGE('',*,*,#18932,.T.);
#27919=ORIENTED_EDGE('',*,*,#18930,.F.);
#27920=ORIENTED_EDGE('',*,*,#18928,.F.);
#27921=ORIENTED_EDGE('',*,*,#18936,.T.);
#27922=ORIENTED_EDGE('',*,*,#19180,.F.);
#27923=ORIENTED_EDGE('',*,*,#19151,.T.);
#27924=ORIENTED_EDGE('',*,*,#19153,.F.);
#27925=ORIENTED_EDGE('',*,*,#18944,.T.);
#27926=ORIENTED_EDGE('',*,*,#19186,.F.);
#27927=ORIENTED_EDGE('',*,*,#19187,.T.);
#27928=ORIENTED_EDGE('',*,*,#18927,.T.);
#27929=ORIENTED_EDGE('',*,*,#19187,.F.);
#27930=ORIENTED_EDGE('',*,*,#19188,.F.);
#27931=ORIENTED_EDGE('',*,*,#19189,.T.);
#27932=ORIENTED_EDGE('',*,*,#19186,.T.);
#27933=ORIENTED_EDGE('',*,*,#19189,.F.);
#27934=ORIENTED_EDGE('',*,*,#19190,.F.);
#27935=ORIENTED_EDGE('',*,*,#19188,.T.);
#27936=ORIENTED_EDGE('',*,*,#18974,.F.);
#27937=ORIENTED_EDGE('',*,*,#19191,.T.);
#27938=ORIENTED_EDGE('',*,*,#19190,.T.);
#27939=ORIENTED_EDGE('',*,*,#19191,.F.);
#27940=ORIENTED_EDGE('',*,*,#18925,.F.);
#28832=PLANE('',#33161);
#28833=PLANE('',#33163);
#28834=PLANE('',#33167);
#28835=PLANE('',#33203);
#28836=PLANE('',#33207);
#28837=PLANE('',#33210);
#28838=PLANE('',#33214);
#28839=PLANE('',#33217);
#28840=PLANE('',#33221);
#28841=PLANE('',#33224);
#28842=PLANE('',#33228);
#28843=PLANE('',#33231);
#28844=PLANE('',#33235);
#28845=PLANE('',#33238);
#28846=PLANE('',#33242);
#28847=PLANE('',#33245);
#28848=PLANE('',#33249);
#28849=PLANE('',#33252);
#28850=PLANE('',#33256);
#28851=PLANE('',#33259);
#28852=PLANE('',#33263);
#28853=PLANE('',#33266);
#28854=PLANE('',#33270);
#28855=PLANE('',#33273);
#28856=PLANE('',#33277);
#28857=PLANE('',#33280);
#28858=PLANE('',#33284);
#28859=PLANE('',#33287);
#28860=PLANE('',#33291);
#28861=PLANE('',#33294);
#28862=PLANE('',#33298);
#28863=PLANE('',#33299);
#28864=PLANE('',#33300);
#28865=PLANE('',#33301);
#28866=PLANE('',#33302);
#28867=PLANE('',#33303);
#28868=PLANE('',#33304);
#28869=PLANE('',#33305);
#28870=PLANE('',#33306);
#28871=PLANE('',#33307);
#28872=PLANE('',#33308);
#28873=PLANE('',#33310);
#28874=PLANE('',#33311);
#28875=PLANE('',#33312);
#28876=PLANE('',#33313);
#28877=PLANE('',#33314);
#28878=PLANE('',#33315);
#28879=PLANE('',#33316);
#28880=PLANE('',#33317);
#28881=PLANE('',#33318);
#28882=PLANE('',#33319);
#28883=PLANE('',#33320);
#28884=PLANE('',#33321);
#28885=PLANE('',#33322);
#28886=PLANE('',#33323);
#28887=PLANE('',#33324);
#28888=PLANE('',#33325);
#28889=PLANE('',#33326);
#28890=PLANE('',#33327);
#28891=PLANE('',#33328);
#28892=PLANE('',#33334);
#28893=PLANE('',#33337);
#30533=ADVANCED_FACE('',(#5205),#2063,.F.);
#30534=ADVANCED_FACE('',(#5206),#1003,.F.);
#30535=ADVANCED_FACE('',(#5207,#3573),#28832,.T.);
#30536=ADVANCED_FACE('',(#5208),#28833,.T.);
#30537=ADVANCED_FACE('',(#5209),#1004,.F.);
#30538=ADVANCED_FACE('',(#5210),#28834,.T.);
#30539=ADVANCED_FACE('',(#5211),#2064,.T.);
#30540=ADVANCED_FACE('',(#5212),#1005,.T.);
#30541=ADVANCED_FACE('',(#5213),#28835,.T.);
#30542=ADVANCED_FACE('',(#5214),#1006,.F.);
#30543=ADVANCED_FACE('',(#5215),#28836,.T.);
#30544=ADVANCED_FACE('',(#5216),#2065,.T.);
#30545=ADVANCED_FACE('',(#5217),#28837,.T.);
#30546=ADVANCED_FACE('',(#5218),#1007,.F.);
#30547=ADVANCED_FACE('',(#5219),#28838,.T.);
#30548=ADVANCED_FACE('',(#5220),#2066,.T.);
#30549=ADVANCED_FACE('',(#5221),#28839,.T.);
#30550=ADVANCED_FACE('',(#5222),#1008,.F.);
#30551=ADVANCED_FACE('',(#5223),#28840,.T.);
#30552=ADVANCED_FACE('',(#5224),#2067,.T.);
#30553=ADVANCED_FACE('',(#5225),#28841,.T.);
#30554=ADVANCED_FACE('',(#5226),#1009,.F.);
#30555=ADVANCED_FACE('',(#5227),#28842,.T.);
#30556=ADVANCED_FACE('',(#5228),#2068,.T.);
#30557=ADVANCED_FACE('',(#5229),#28843,.T.);
#30558=ADVANCED_FACE('',(#5230),#1010,.F.);
#30559=ADVANCED_FACE('',(#5231),#28844,.T.);
#30560=ADVANCED_FACE('',(#5232),#2069,.T.);
#30561=ADVANCED_FACE('',(#5233),#28845,.T.);
#30562=ADVANCED_FACE('',(#5234),#1011,.F.);
#30563=ADVANCED_FACE('',(#5235),#28846,.T.);
#30564=ADVANCED_FACE('',(#5236),#2070,.T.);
#30565=ADVANCED_FACE('',(#5237),#28847,.T.);
#30566=ADVANCED_FACE('',(#5238),#1012,.F.);
#30567=ADVANCED_FACE('',(#5239),#28848,.T.);
#30568=ADVANCED_FACE('',(#5240),#2071,.T.);
#30569=ADVANCED_FACE('',(#5241),#28849,.T.);
#30570=ADVANCED_FACE('',(#5242),#1013,.F.);
#30571=ADVANCED_FACE('',(#5243),#28850,.T.);
#30572=ADVANCED_FACE('',(#5244),#2072,.T.);
#30573=ADVANCED_FACE('',(#5245),#28851,.T.);
#30574=ADVANCED_FACE('',(#5246),#1014,.F.);
#30575=ADVANCED_FACE('',(#5247),#28852,.T.);
#30576=ADVANCED_FACE('',(#5248),#2073,.T.);
#30577=ADVANCED_FACE('',(#5249),#28853,.T.);
#30578=ADVANCED_FACE('',(#5250),#1015,.F.);
#30579=ADVANCED_FACE('',(#5251),#28854,.T.);
#30580=ADVANCED_FACE('',(#5252),#2074,.T.);
#30581=ADVANCED_FACE('',(#5253),#28855,.T.);
#30582=ADVANCED_FACE('',(#5254),#1016,.F.);
#30583=ADVANCED_FACE('',(#5255),#28856,.T.);
#30584=ADVANCED_FACE('',(#5256),#2075,.T.);
#30585=ADVANCED_FACE('',(#5257),#28857,.T.);
#30586=ADVANCED_FACE('',(#5258),#1017,.F.);
#30587=ADVANCED_FACE('',(#5259),#28858,.T.);
#30588=ADVANCED_FACE('',(#5260),#2076,.T.);
#30589=ADVANCED_FACE('',(#5261),#28859,.T.);
#30590=ADVANCED_FACE('',(#5262),#1018,.F.);
#30591=ADVANCED_FACE('',(#5263),#28860,.T.);
#30592=ADVANCED_FACE('',(#5264),#2077,.T.);
#30593=ADVANCED_FACE('',(#5265),#28861,.T.);
#30594=ADVANCED_FACE('',(#5266),#1019,.F.);
#30595=ADVANCED_FACE('',(#5267),#28862,.T.);
#30596=ADVANCED_FACE('',(#5268),#28863,.T.);
#30597=ADVANCED_FACE('',(#5269),#28864,.T.);
#30598=ADVANCED_FACE('',(#5270),#28865,.T.);
#30599=ADVANCED_FACE('',(#5271),#28866,.T.);
#30600=ADVANCED_FACE('',(#5272),#28867,.T.);
#30601=ADVANCED_FACE('',(#5273),#28868,.T.);
#30602=ADVANCED_FACE('',(#5274),#28869,.F.);
#30603=ADVANCED_FACE('',(#5275),#28870,.F.);
#30604=ADVANCED_FACE('',(#5276),#28871,.F.);
#30605=ADVANCED_FACE('',(#5277,#3574),#28872,.T.);
#30606=ADVANCED_FACE('',(#5278),#28873,.F.);
#30607=ADVANCED_FACE('',(#5279),#28874,.F.);
#30608=ADVANCED_FACE('',(#5280),#28875,.F.);
#30609=ADVANCED_FACE('',(#5281),#28876,.F.);
#30610=ADVANCED_FACE('',(#5282),#28877,.T.);
#30611=ADVANCED_FACE('',(#5283),#28878,.T.);
#30612=ADVANCED_FACE('',(#5284),#28879,.T.);
#30613=ADVANCED_FACE('',(#5285),#28880,.T.);
#30614=ADVANCED_FACE('',(#5286),#28881,.T.);
#30615=ADVANCED_FACE('',(#5287),#28882,.T.);
#30616=ADVANCED_FACE('',(#5288),#28883,.T.);
#30617=ADVANCED_FACE('',(#5289),#28884,.T.);
#30618=ADVANCED_FACE('',(#5290),#28885,.T.);
#30619=ADVANCED_FACE('',(#5291),#28886,.T.);
#30620=ADVANCED_FACE('',(#5292),#28887,.T.);
#30621=ADVANCED_FACE('',(#5293),#28888,.T.);
#30622=ADVANCED_FACE('',(#5294),#28889,.T.);
#30623=ADVANCED_FACE('',(#5295),#28890,.T.);
#30624=ADVANCED_FACE('',(#5296),#28891,.T.);
#30625=ADVANCED_FACE('',(#5297),#2078,.T.);
#30626=ADVANCED_FACE('',(#5298),#2079,.T.);
#30627=ADVANCED_FACE('',(#5299),#1020,.T.);
#30628=ADVANCED_FACE('',(#5300,#3575),#28892,.T.);
#30629=ADVANCED_FACE('',(#5301),#2080,.T.);
#30630=ADVANCED_FACE('',(#5302),#28893,.T.);
#30678=CLOSED_SHELL('',(#30533,#30534,#30535,#30536,#30537,#30538,#30539,
#30540,#30541,#30542,#30543,#30544,#30545,#30546,#30547,#30548,#30549,#30550,
#30551,#30552,#30553,#30554,#30555,#30556,#30557,#30558,#30559,#30560,#30561,
#30562,#30563,#30564,#30565,#30566,#30567,#30568,#30569,#30570,#30571,#30572,
#30573,#30574,#30575,#30576,#30577,#30578,#30579,#30580,#30581,#30582,#30583,
#30584,#30585,#30586,#30587,#30588,#30589,#30590,#30591,#30592,#30593,#30594,
#30595,#30596,#30597,#30598,#30599,#30600,#30601,#30602,#30603,#30604,#30605,
#30606,#30607,#30608,#30609,#30610,#30611,#30612,#30613,#30614,#30615,#30616,
#30617,#30618,#30619,#30620,#30621,#30622,#30623,#30624,#30625,#30626,#30627,
#30628,#30629,#30630));
#33154=AXIS2_PLACEMENT_3D('',#80263,#40088,#40089);
#33155=AXIS2_PLACEMENT_3D('',#80264,#40090,#40091);
#33156=AXIS2_PLACEMENT_3D('',#80266,#40092,#40093);
#33157=AXIS2_PLACEMENT_3D('',#80270,#40095,#40096);
#33158=AXIS2_PLACEMENT_3D('',#80271,#40097,#40098);
#33159=AXIS2_PLACEMENT_3D('',#80272,#40099,#40100);
#33160=AXIS2_PLACEMENT_3D('',#80274,#40101,#40102);
#33161=AXIS2_PLACEMENT_3D('',#80276,#40104,#40105);
#33162=AXIS2_PLACEMENT_3D('',#80278,#40106,#40107);
#33163=AXIS2_PLACEMENT_3D('',#80279,#40108,#40109);
#33164=AXIS2_PLACEMENT_3D('',#80290,#40113,#40114);
#33165=AXIS2_PLACEMENT_3D('',#80292,#40115,#40116);
#33166=AXIS2_PLACEMENT_3D('',#80303,#40118,#40119);
#33167=AXIS2_PLACEMENT_3D('',#80310,#40120,#40121);
#33168=AXIS2_PLACEMENT_3D('',#80318,#40124,#40125);
#33169=AXIS2_PLACEMENT_3D('',#80320,#40126,#40127);
#33170=AXIS2_PLACEMENT_3D('',#80332,#40128,#40129);
#33171=AXIS2_PLACEMENT_3D('',#80333,#40130,#40131);
#33172=AXIS2_PLACEMENT_3D('',#80335,#40132,#40133);
#33173=AXIS2_PLACEMENT_3D('',#80339,#40135,#40136);
#33174=AXIS2_PLACEMENT_3D('',#80343,#40138,#40139);
#33175=AXIS2_PLACEMENT_3D('',#80347,#40141,#40142);
#33176=AXIS2_PLACEMENT_3D('',#80351,#40144,#40145);
#33177=AXIS2_PLACEMENT_3D('',#80355,#40147,#40148);
#33178=AXIS2_PLACEMENT_3D('',#80359,#40150,#40151);
#33179=AXIS2_PLACEMENT_3D('',#80363,#40153,#40154);
#33180=AXIS2_PLACEMENT_3D('',#80367,#40156,#40157);
#33181=AXIS2_PLACEMENT_3D('',#80371,#40159,#40160);
#33182=AXIS2_PLACEMENT_3D('',#80375,#40162,#40163);
#33183=AXIS2_PLACEMENT_3D('',#80379,#40165,#40166);
#33184=AXIS2_PLACEMENT_3D('',#80383,#40168,#40169);
#33185=AXIS2_PLACEMENT_3D('',#80387,#40171,#40172);
#33186=AXIS2_PLACEMENT_3D('',#80391,#40174,#40175);
#33187=AXIS2_PLACEMENT_3D('',#80394,#40177,#40178);
#33188=AXIS2_PLACEMENT_3D('',#80396,#40179,#40180);
#33189=AXIS2_PLACEMENT_3D('',#80400,#40182,#40183);
#33190=AXIS2_PLACEMENT_3D('',#80404,#40185,#40186);
#33191=AXIS2_PLACEMENT_3D('',#80408,#40188,#40189);
#33192=AXIS2_PLACEMENT_3D('',#80412,#40191,#40192);
#33193=AXIS2_PLACEMENT_3D('',#80416,#40194,#40195);
#33194=AXIS2_PLACEMENT_3D('',#80420,#40197,#40198);
#33195=AXIS2_PLACEMENT_3D('',#80424,#40200,#40201);
#33196=AXIS2_PLACEMENT_3D('',#80428,#40203,#40204);
#33197=AXIS2_PLACEMENT_3D('',#80432,#40206,#40207);
#33198=AXIS2_PLACEMENT_3D('',#80436,#40209,#40210);
#33199=AXIS2_PLACEMENT_3D('',#80440,#40212,#40213);
#33200=AXIS2_PLACEMENT_3D('',#80444,#40215,#40216);
#33201=AXIS2_PLACEMENT_3D('',#80448,#40218,#40219);
#33202=AXIS2_PLACEMENT_3D('',#80450,#40221,#40222);
#33203=AXIS2_PLACEMENT_3D('',#80451,#40223,#40224);
#33204=AXIS2_PLACEMENT_3D('',#80455,#40227,#40228);
#33205=AXIS2_PLACEMENT_3D('',#80457,#40229,#40230);
#33206=AXIS2_PLACEMENT_3D('',#80467,#40232,#40233);
#33207=AXIS2_PLACEMENT_3D('',#80468,#40234,#40235);
#33208=AXIS2_PLACEMENT_3D('',#80473,#40237,#40238);
#33209=AXIS2_PLACEMENT_3D('',#80485,#40239,#40240);
#33210=AXIS2_PLACEMENT_3D('',#80486,#40241,#40242);
#33211=AXIS2_PLACEMENT_3D('',#80490,#40245,#40246);
#33212=AXIS2_PLACEMENT_3D('',#80492,#40247,#40248);
#33213=AXIS2_PLACEMENT_3D('',#80502,#40250,#40251);
#33214=AXIS2_PLACEMENT_3D('',#80503,#40252,#40253);
#33215=AXIS2_PLACEMENT_3D('',#80508,#40255,#40256);
#33216=AXIS2_PLACEMENT_3D('',#80520,#40257,#40258);
#33217=AXIS2_PLACEMENT_3D('',#80521,#40259,#40260);
#33218=AXIS2_PLACEMENT_3D('',#80525,#40263,#40264);
#33219=AXIS2_PLACEMENT_3D('',#80527,#40265,#40266);
#33220=AXIS2_PLACEMENT_3D('',#80537,#40268,#40269);
#33221=AXIS2_PLACEMENT_3D('',#80538,#40270,#40271);
#33222=AXIS2_PLACEMENT_3D('',#80543,#40273,#40274);
#33223=AXIS2_PLACEMENT_3D('',#80555,#40275,#40276);
#33224=AXIS2_PLACEMENT_3D('',#80556,#40277,#40278);
#33225=AXIS2_PLACEMENT_3D('',#80560,#40281,#40282);
#33226=AXIS2_PLACEMENT_3D('',#80562,#40283,#40284);
#33227=AXIS2_PLACEMENT_3D('',#80572,#40286,#40287);
#33228=AXIS2_PLACEMENT_3D('',#80573,#40288,#40289);
#33229=AXIS2_PLACEMENT_3D('',#80578,#40291,#40292);
#33230=AXIS2_PLACEMENT_3D('',#80590,#40293,#40294);
#33231=AXIS2_PLACEMENT_3D('',#80591,#40295,#40296);
#33232=AXIS2_PLACEMENT_3D('',#80595,#40299,#40300);
#33233=AXIS2_PLACEMENT_3D('',#80597,#40301,#40302);
#33234=AXIS2_PLACEMENT_3D('',#80607,#40304,#40305);
#33235=AXIS2_PLACEMENT_3D('',#80608,#40306,#40307);
#33236=AXIS2_PLACEMENT_3D('',#80613,#40309,#40310);
#33237=AXIS2_PLACEMENT_3D('',#80625,#40311,#40312);
#33238=AXIS2_PLACEMENT_3D('',#80626,#40313,#40314);
#33239=AXIS2_PLACEMENT_3D('',#80630,#40317,#40318);
#33240=AXIS2_PLACEMENT_3D('',#80632,#40319,#40320);
#33241=AXIS2_PLACEMENT_3D('',#80642,#40322,#40323);
#33242=AXIS2_PLACEMENT_3D('',#80643,#40324,#40325);
#33243=AXIS2_PLACEMENT_3D('',#80648,#40327,#40328);
#33244=AXIS2_PLACEMENT_3D('',#80660,#40329,#40330);
#33245=AXIS2_PLACEMENT_3D('',#80661,#40331,#40332);
#33246=AXIS2_PLACEMENT_3D('',#80665,#40335,#40336);
#33247=AXIS2_PLACEMENT_3D('',#80667,#40337,#40338);
#33248=AXIS2_PLACEMENT_3D('',#80677,#40340,#40341);
#33249=AXIS2_PLACEMENT_3D('',#80678,#40342,#40343);
#33250=AXIS2_PLACEMENT_3D('',#80683,#40345,#40346);
#33251=AXIS2_PLACEMENT_3D('',#80695,#40347,#40348);
#33252=AXIS2_PLACEMENT_3D('',#80696,#40349,#40350);
#33253=AXIS2_PLACEMENT_3D('',#80700,#40353,#40354);
#33254=AXIS2_PLACEMENT_3D('',#80702,#40355,#40356);
#33255=AXIS2_PLACEMENT_3D('',#80712,#40358,#40359);
#33256=AXIS2_PLACEMENT_3D('',#80713,#40360,#40361);
#33257=AXIS2_PLACEMENT_3D('',#80718,#40363,#40364);
#33258=AXIS2_PLACEMENT_3D('',#80730,#40365,#40366);
#33259=AXIS2_PLACEMENT_3D('',#80731,#40367,#40368);
#33260=AXIS2_PLACEMENT_3D('',#80735,#40371,#40372);
#33261=AXIS2_PLACEMENT_3D('',#80737,#40373,#40374);
#33262=AXIS2_PLACEMENT_3D('',#80747,#40376,#40377);
#33263=AXIS2_PLACEMENT_3D('',#80748,#40378,#40379);
#33264=AXIS2_PLACEMENT_3D('',#80753,#40381,#40382);
#33265=AXIS2_PLACEMENT_3D('',#80765,#40383,#40384);
#33266=AXIS2_PLACEMENT_3D('',#80766,#40385,#40386);
#33267=AXIS2_PLACEMENT_3D('',#80770,#40389,#40390);
#33268=AXIS2_PLACEMENT_3D('',#80772,#40391,#40392);
#33269=AXIS2_PLACEMENT_3D('',#80782,#40394,#40395);
#33270=AXIS2_PLACEMENT_3D('',#80783,#40396,#40397);
#33271=AXIS2_PLACEMENT_3D('',#80788,#40399,#40400);
#33272=AXIS2_PLACEMENT_3D('',#80800,#40401,#40402);
#33273=AXIS2_PLACEMENT_3D('',#80801,#40403,#40404);
#33274=AXIS2_PLACEMENT_3D('',#80805,#40407,#40408);
#33275=AXIS2_PLACEMENT_3D('',#80807,#40409,#40410);
#33276=AXIS2_PLACEMENT_3D('',#80817,#40412,#40413);
#33277=AXIS2_PLACEMENT_3D('',#80818,#40414,#40415);
#33278=AXIS2_PLACEMENT_3D('',#80823,#40417,#40418);
#33279=AXIS2_PLACEMENT_3D('',#80835,#40419,#40420);
#33280=AXIS2_PLACEMENT_3D('',#80836,#40421,#40422);
#33281=AXIS2_PLACEMENT_3D('',#80840,#40425,#40426);
#33282=AXIS2_PLACEMENT_3D('',#80842,#40427,#40428);
#33283=AXIS2_PLACEMENT_3D('',#80852,#40430,#40431);
#33284=AXIS2_PLACEMENT_3D('',#80853,#40432,#40433);
#33285=AXIS2_PLACEMENT_3D('',#80858,#40435,#40436);
#33286=AXIS2_PLACEMENT_3D('',#80870,#40437,#40438);
#33287=AXIS2_PLACEMENT_3D('',#80871,#40439,#40440);
#33288=AXIS2_PLACEMENT_3D('',#80875,#40443,#40444);
#33289=AXIS2_PLACEMENT_3D('',#80877,#40445,#40446);
#33290=AXIS2_PLACEMENT_3D('',#80887,#40448,#40449);
#33291=AXIS2_PLACEMENT_3D('',#80888,#40450,#40451);
#33292=AXIS2_PLACEMENT_3D('',#80893,#40453,#40454);
#33293=AXIS2_PLACEMENT_3D('',#80905,#40455,#40456);
#33294=AXIS2_PLACEMENT_3D('',#80906,#40457,#40458);
#33295=AXIS2_PLACEMENT_3D('',#80910,#40461,#40462);
#33296=AXIS2_PLACEMENT_3D('',#80912,#40463,#40464);
#33297=AXIS2_PLACEMENT_3D('',#80922,#40466,#40467);
#33298=AXIS2_PLACEMENT_3D('',#80923,#40468,#40469);
#33299=AXIS2_PLACEMENT_3D('',#80928,#40471,#40472);
#33300=AXIS2_PLACEMENT_3D('',#80937,#40477,#40478);
#33301=AXIS2_PLACEMENT_3D('',#80943,#40482,#40483);
#33302=AXIS2_PLACEMENT_3D('',#80952,#40488,#40489);
#33303=AXIS2_PLACEMENT_3D('',#80958,#40493,#40494);
#33304=AXIS2_PLACEMENT_3D('',#80961,#40497,#40498);
#33305=AXIS2_PLACEMENT_3D('',#80964,#40501,#40502);
#33306=AXIS2_PLACEMENT_3D('',#80970,#40506,#40507);
#33307=AXIS2_PLACEMENT_3D('',#80974,#40510,#40511);
#33308=AXIS2_PLACEMENT_3D('',#80978,#40514,#40515);
#33309=AXIS2_PLACEMENT_3D('',#80979,#40516,#40517);
#33310=AXIS2_PLACEMENT_3D('',#80980,#40518,#40519);
#33311=AXIS2_PLACEMENT_3D('',#80984,#40522,#40523);
#33312=AXIS2_PLACEMENT_3D('',#80988,#40526,#40527);
#33313=AXIS2_PLACEMENT_3D('',#80990,#40529,#40530);
#33314=AXIS2_PLACEMENT_3D('',#80991,#40531,#40532);
#33315=AXIS2_PLACEMENT_3D('',#80992,#40533,#40534);
#33316=AXIS2_PLACEMENT_3D('',#80993,#40535,#40536);
#33317=AXIS2_PLACEMENT_3D('',#80994,#40537,#40538);
#33318=AXIS2_PLACEMENT_3D('',#80995,#40539,#40540);
#33319=AXIS2_PLACEMENT_3D('',#80996,#40541,#40542);
#33320=AXIS2_PLACEMENT_3D('',#80997,#40543,#40544);
#33321=AXIS2_PLACEMENT_3D('',#80998,#40545,#40546);
#33322=AXIS2_PLACEMENT_3D('',#80999,#40547,#40548);
#33323=AXIS2_PLACEMENT_3D('',#81000,#40549,#40550);
#33324=AXIS2_PLACEMENT_3D('',#81001,#40551,#40552);
#33325=AXIS2_PLACEMENT_3D('',#81002,#40553,#40554);
#33326=AXIS2_PLACEMENT_3D('',#81003,#40555,#40556);
#33327=AXIS2_PLACEMENT_3D('',#81004,#40557,#40558);
#33328=AXIS2_PLACEMENT_3D('',#81005,#40559,#40560);
#33329=AXIS2_PLACEMENT_3D('',#81006,#40561,#40562);
#33330=AXIS2_PLACEMENT_3D('',#81007,#40563,#40564);
#33331=AXIS2_PLACEMENT_3D('',#81009,#40565,#40566);
#33332=AXIS2_PLACEMENT_3D('',#81011,#40568,#40569);
#33333=AXIS2_PLACEMENT_3D('',#81013,#40570,#40571);
#33334=AXIS2_PLACEMENT_3D('',#81015,#40573,#40574);
#33335=AXIS2_PLACEMENT_3D('',#81017,#40575,#40576);
#33336=AXIS2_PLACEMENT_3D('',#81018,#40577,#40578);
#33337=AXIS2_PLACEMENT_3D('',#81020,#40580,#40581);
#40088=DIRECTION('axis',(0.,0.,1.));
#40089=DIRECTION('refdir',(1.,0.,0.));
#40090=DIRECTION('center_axis',(-1.,0.,0.));
#40091=DIRECTION('ref_axis',(0.,-1.,0.));
#40092=DIRECTION('center_axis',(-1.,0.,0.));
#40093=DIRECTION('ref_axis',(0.,-1.,0.));
#40094=DIRECTION('',(0.707106781186546,-0.707106781186549,8.65956056235495E-17));
#40095=DIRECTION('center_axis',(1.,0.,0.));
#40096=DIRECTION('ref_axis',(0.,-1.,0.));
#40097=DIRECTION('center_axis',(1.,0.,0.));
#40098=DIRECTION('ref_axis',(0.,-1.,0.));
#40099=DIRECTION('center_axis',(1.,0.,0.));
#40100=DIRECTION('ref_axis',(0.,1.,0.));
#40101=DIRECTION('center_axis',(1.,0.,0.));
#40102=DIRECTION('ref_axis',(0.,0.,-1.));
#40103=DIRECTION('',(-1.,0.,0.));
#40104=DIRECTION('center_axis',(-1.,0.,0.));
#40105=DIRECTION('ref_axis',(0.,0.,1.));
#40106=DIRECTION('center_axis',(1.,0.,0.));
#40107=DIRECTION('ref_axis',(0.,0.,-1.));
#40108=DIRECTION('center_axis',(0.,0.92942454284145,0.369012220887006));
#40109=DIRECTION('ref_axis',(0.,-0.369012220887006,0.929424542841451));
#40110=DIRECTION('',(-1.,0.,0.));
#40111=DIRECTION('',(0.,0.369012220887006,-0.929424542841451));
#40112=DIRECTION('',(1.,0.,0.));
#40113=DIRECTION('center_axis',(1.,0.,0.));
#40114=DIRECTION('ref_axis',(0.,0.,-1.));
#40115=DIRECTION('center_axis',(1.,0.,0.));
#40116=DIRECTION('ref_axis',(0.,0.,-1.));
#40117=DIRECTION('',(-1.,0.,0.));
#40118=DIRECTION('center_axis',(-1.,0.,0.));
#40119=DIRECTION('ref_axis',(0.,0.,-1.));
#40120=DIRECTION('center_axis',(0.,0.92942454284145,-0.369012220887006));
#40121=DIRECTION('ref_axis',(0.,0.369012220887006,0.929424542841451));
#40122=DIRECTION('',(0.,-0.369012220887006,-0.929424542841451));
#40123=DIRECTION('',(1.,0.,0.));
#40124=DIRECTION('center_axis',(-1.,0.,0.));
#40125=DIRECTION('ref_axis',(0.,1.,0.));
#40126=DIRECTION('center_axis',(1.,0.,0.));
#40127=DIRECTION('ref_axis',(0.,0.,-1.));
#40128=DIRECTION('center_axis',(1.,0.,0.));
#40129=DIRECTION('ref_axis',(0.,0.,-1.));
#40130=DIRECTION('center_axis',(1.,0.,0.));
#40131=DIRECTION('ref_axis',(0.,1.,0.));
#40132=DIRECTION('center_axis',(1.,0.,0.));
#40133=DIRECTION('ref_axis',(0.,0.,-1.));
#40134=DIRECTION('',(1.,0.,0.));
#40135=DIRECTION('center_axis',(-1.,0.,0.));
#40136=DIRECTION('ref_axis',(0.,1.,0.));
#40137=DIRECTION('',(-1.,0.,0.));
#40138=DIRECTION('center_axis',(1.,0.,0.));
#40139=DIRECTION('ref_axis',(0.,0.,-1.));
#40140=DIRECTION('',(1.,0.,0.));
#40141=DIRECTION('center_axis',(-1.,0.,0.));
#40142=DIRECTION('ref_axis',(0.,1.,0.));
#40143=DIRECTION('',(-1.,0.,0.));
#40144=DIRECTION('center_axis',(1.,0.,0.));
#40145=DIRECTION('ref_axis',(0.,0.,-1.));
#40146=DIRECTION('',(1.,0.,0.));
#40147=DIRECTION('center_axis',(-1.,0.,0.));
#40148=DIRECTION('ref_axis',(0.,1.,0.));
#40149=DIRECTION('',(-1.,0.,0.));
#40150=DIRECTION('center_axis',(1.,0.,0.));
#40151=DIRECTION('ref_axis',(0.,0.,-1.));
#40152=DIRECTION('',(1.,0.,0.));
#40153=DIRECTION('center_axis',(-1.,0.,0.));
#40154=DIRECTION('ref_axis',(0.,1.,0.));
#40155=DIRECTION('',(-1.,0.,0.));
#40156=DIRECTION('center_axis',(1.,0.,0.));
#40157=DIRECTION('ref_axis',(0.,0.,-1.));
#40158=DIRECTION('',(1.,0.,0.));
#40159=DIRECTION('center_axis',(-1.,0.,0.));
#40160=DIRECTION('ref_axis',(0.,1.,0.));
#40161=DIRECTION('',(-1.,0.,0.));
#40162=DIRECTION('center_axis',(1.,0.,0.));
#40163=DIRECTION('ref_axis',(0.,0.,-1.));
#40164=DIRECTION('',(1.,0.,0.));
#40165=DIRECTION('center_axis',(-1.,0.,0.));
#40166=DIRECTION('ref_axis',(0.,1.,0.));
#40167=DIRECTION('',(-1.,0.,0.));
#40168=DIRECTION('center_axis',(1.,0.,0.));
#40169=DIRECTION('ref_axis',(0.,0.,-1.));
#40170=DIRECTION('',(1.,0.,0.));
#40171=DIRECTION('center_axis',(-1.,0.,0.));
#40172=DIRECTION('ref_axis',(0.,1.,0.));
#40173=DIRECTION('',(-1.,0.,0.));
#40174=DIRECTION('center_axis',(1.,0.,0.));
#40175=DIRECTION('ref_axis',(0.,0.,-1.));
#40176=DIRECTION('',(-1.,0.,0.));
#40177=DIRECTION('center_axis',(1.,0.,0.));
#40178=DIRECTION('ref_axis',(0.,0.,-1.));
#40179=DIRECTION('center_axis',(1.,0.,0.));
#40180=DIRECTION('ref_axis',(0.,0.,-1.));
#40181=DIRECTION('',(1.,0.,0.));
#40182=DIRECTION('center_axis',(-1.,0.,0.));
#40183=DIRECTION('ref_axis',(0.,1.,0.));
#40184=DIRECTION('',(-1.,0.,0.));
#40185=DIRECTION('center_axis',(1.,0.,0.));
#40186=DIRECTION('ref_axis',(0.,0.,-1.));
#40187=DIRECTION('',(1.,0.,0.));
#40188=DIRECTION('center_axis',(-1.,0.,0.));
#40189=DIRECTION('ref_axis',(0.,1.,0.));
#40190=DIRECTION('',(-1.,0.,0.));
#40191=DIRECTION('center_axis',(1.,0.,0.));
#40192=DIRECTION('ref_axis',(0.,0.,-1.));
#40193=DIRECTION('',(1.,0.,0.));
#40194=DIRECTION('center_axis',(-1.,0.,0.));
#40195=DIRECTION('ref_axis',(0.,1.,0.));
#40196=DIRECTION('',(-1.,0.,0.));
#40197=DIRECTION('center_axis',(1.,0.,0.));
#40198=DIRECTION('ref_axis',(0.,0.,-1.));
#40199=DIRECTION('',(1.,0.,0.));
#40200=DIRECTION('center_axis',(-1.,0.,0.));
#40201=DIRECTION('ref_axis',(0.,1.,0.));
#40202=DIRECTION('',(-1.,0.,0.));
#40203=DIRECTION('center_axis',(1.,0.,0.));
#40204=DIRECTION('ref_axis',(0.,0.,-1.));
#40205=DIRECTION('',(1.,0.,0.));
#40206=DIRECTION('center_axis',(-1.,0.,0.));
#40207=DIRECTION('ref_axis',(0.,1.,0.));
#40208=DIRECTION('',(-1.,0.,0.));
#40209=DIRECTION('center_axis',(1.,0.,0.));
#40210=DIRECTION('ref_axis',(0.,0.,-1.));
#40211=DIRECTION('',(1.,0.,0.));
#40212=DIRECTION('center_axis',(-1.,0.,0.));
#40213=DIRECTION('ref_axis',(0.,1.,0.));
#40214=DIRECTION('',(-1.,0.,0.));
#40215=DIRECTION('center_axis',(1.,0.,0.));
#40216=DIRECTION('ref_axis',(0.,0.,-1.));
#40217=DIRECTION('',(1.,0.,0.));
#40218=DIRECTION('center_axis',(-1.,0.,0.));
#40219=DIRECTION('ref_axis',(0.,1.,0.));
#40220=DIRECTION('',(-1.,0.,0.));
#40221=DIRECTION('center_axis',(-1.,0.,0.));
#40222=DIRECTION('ref_axis',(0.,1.,0.));
#40223=DIRECTION('center_axis',(0.,0.698980777356835,0.715140456753522));
#40224=DIRECTION('ref_axis',(1.,0.,0.));
#40225=DIRECTION('',(0.,0.715140456753521,-0.698980777356835));
#40226=DIRECTION('',(1.,0.,0.));
#40227=DIRECTION('center_axis',(1.,0.,0.));
#40228=DIRECTION('ref_axis',(0.,0.4067366430758,-0.913545457642601));
#40229=DIRECTION('center_axis',(1.,0.,0.));
#40230=DIRECTION('ref_axis',(0.,0.4067366430758,-0.913545457642601));
#40231=DIRECTION('',(-1.,0.,0.));
#40232=DIRECTION('center_axis',(-1.,0.,0.));
#40233=DIRECTION('ref_axis',(0.,0.4067366430758,-0.913545457642601));
#40234=DIRECTION('center_axis',(0.,0.999162361311885,0.0409215803416579));
#40235=DIRECTION('ref_axis',(0.,-0.0409215803416579,0.999162361311885));
#40236=DIRECTION('',(0.,0.0409215803416579,-0.999162361311885));
#40237=DIRECTION('center_axis',(-1.,0.,0.));
#40238=DIRECTION('ref_axis',(0.,1.,0.));
#40239=DIRECTION('center_axis',(1.,0.,0.));
#40240=DIRECTION('ref_axis',(0.,0.,-1.));
#40241=DIRECTION('center_axis',(0.,0.347676885426204,0.937614410800268));
#40242=DIRECTION('ref_axis',(1.,0.,0.));
#40243=DIRECTION('',(0.,0.937614410800268,-0.347676885426204));
#40244=DIRECTION('',(1.,0.,0.));
#40245=DIRECTION('center_axis',(1.,0.,0.));
#40246=DIRECTION('ref_axis',(0.,0.743144825477394,-0.669130606358858));
#40247=DIRECTION('center_axis',(1.,0.,0.));
#40248=DIRECTION('ref_axis',(0.,0.743144825477394,-0.669130606358858));
#40249=DIRECTION('',(-1.,0.,0.));
#40250=DIRECTION('center_axis',(-1.,0.,0.));
#40251=DIRECTION('ref_axis',(0.,0.743144825477394,-0.669130606358858));
#40252=DIRECTION('center_axis',(0.,0.896135930406404,0.443779668568366));
#40253=DIRECTION('ref_axis',(0.,-0.443779668568366,0.896135930406404));
#40254=DIRECTION('',(0.,0.443779668568366,-0.896135930406404));
#40255=DIRECTION('center_axis',(-1.,0.,0.));
#40256=DIRECTION('ref_axis',(0.,1.,0.));
#40257=DIRECTION('center_axis',(1.,0.,0.));
#40258=DIRECTION('ref_axis',(0.,0.,-1.));
#40259=DIRECTION('center_axis',(0.,-0.0637434985399573,0.997966315260133));
#40260=DIRECTION('ref_axis',(1.,0.,0.));
#40261=DIRECTION('',(0.,0.997966315260133,0.0637434985399573));
#40262=DIRECTION('',(1.,0.,0.));
#40263=DIRECTION('center_axis',(1.,0.,0.));
#40264=DIRECTION('ref_axis',(0.,0.951056516295154,-0.309016994374947));
#40265=DIRECTION('center_axis',(1.,0.,0.));
#40266=DIRECTION('ref_axis',(0.,0.951056516295154,-0.309016994374947));
#40267=DIRECTION('',(-1.,0.,0.));
#40268=DIRECTION('center_axis',(-1.,0.,0.));
#40269=DIRECTION('ref_axis',(0.,0.951056516295154,-0.309016994374947));
#40270=DIRECTION('center_axis',(0.,0.63815945599431,0.769904220487877));
#40271=DIRECTION('ref_axis',(1.,0.,0.));
#40272=DIRECTION('',(0.,0.769904220487877,-0.63815945599431));
#40273=DIRECTION('center_axis',(-1.,0.,0.));
#40274=DIRECTION('ref_axis',(0.,1.,0.));
#40275=DIRECTION('center_axis',(1.,0.,0.));
#40276=DIRECTION('ref_axis',(0.,0.,-1.));
#40277=DIRECTION('center_axis',(0.,-0.46414205251706,0.885760777572168));
#40278=DIRECTION('ref_axis',(1.,0.,0.));
#40279=DIRECTION('',(0.,0.885760777572168,0.46414205251706));
#40280=DIRECTION('',(1.,0.,0.));
#40281=DIRECTION('center_axis',(1.,0.,0.));
#40282=DIRECTION('ref_axis',(0.,0.994521895368273,0.104528463267653));
#40283=DIRECTION('center_axis',(1.,0.,0.));
#40284=DIRECTION('ref_axis',(0.,0.994521895368273,0.104528463267653));
#40285=DIRECTION('',(-1.,0.,0.));
#40286=DIRECTION('center_axis',(-1.,0.,0.));
#40287=DIRECTION('ref_axis',(0.,0.994521895368273,0.104528463267653));
#40288=DIRECTION('center_axis',(0.,0.269839414144142,0.962905338324773));
#40289=DIRECTION('ref_axis',(1.,0.,0.));
#40290=DIRECTION('',(0.,0.962905338324773,-0.269839414144142));
#40291=DIRECTION('center_axis',(-1.,0.,0.));
#40292=DIRECTION('ref_axis',(0.,1.,0.));
#40293=DIRECTION('center_axis',(1.,0.,0.));
#40294=DIRECTION('ref_axis',(0.,0.,-1.));
#40295=DIRECTION('center_axis',(0.,-0.784286229015789,0.620399154557929));
#40296=DIRECTION('ref_axis',(1.,0.,0.));
#40297=DIRECTION('',(0.,0.620399154557929,0.784286229015789));
#40298=DIRECTION('',(1.,0.,0.));
#40299=DIRECTION('center_axis',(1.,0.,0.));
#40300=DIRECTION('ref_axis',(0.,0.866025403784439,0.5));
#40301=DIRECTION('center_axis',(1.,0.,0.));
#40302=DIRECTION('ref_axis',(0.,0.866025403784439,0.5));
#40303=DIRECTION('',(-1.,0.,0.));
#40304=DIRECTION('center_axis',(-1.,0.,0.));
#40305=DIRECTION('ref_axis',(0.,0.866025403784439,0.5));
#40306=DIRECTION('center_axis',(0.,-0.145138313825661,0.989411375444938));
#40307=DIRECTION('ref_axis',(1.,0.,0.));
#40308=DIRECTION('',(0.,0.989411375444938,0.145138313825661));
#40309=DIRECTION('center_axis',(-1.,0.,0.));
#40310=DIRECTION('ref_axis',(0.,1.,0.));
#40311=DIRECTION('center_axis',(1.,0.,0.));
#40312=DIRECTION('ref_axis',(0.,0.,-1.));
#40313=DIRECTION('center_axis',(0.,-0.968820191500975,0.247764881571245));
#40314=DIRECTION('ref_axis',(0.,-0.247764881571245,-0.968820191500975));
#40315=DIRECTION('',(0.,0.247764881571245,0.968820191500975));
#40316=DIRECTION('',(1.,0.,0.));
#40317=DIRECTION('center_axis',(1.,0.,0.));
#40318=DIRECTION('ref_axis',(0.,0.587785252292473,0.809016994374947));
#40319=DIRECTION('center_axis',(1.,0.,0.));
#40320=DIRECTION('ref_axis',(0.,0.587785252292473,0.809016994374947));
#40321=DIRECTION('',(-1.,0.,0.));
#40322=DIRECTION('center_axis',(-1.,0.,0.));
#40323=DIRECTION('ref_axis',(0.,0.587785252292473,0.809016994374947));
#40324=DIRECTION('center_axis',(0.,-0.535020308794828,0.844839197230507));
#40325=DIRECTION('ref_axis',(1.,0.,0.));
#40326=DIRECTION('',(0.,0.844839197230507,0.535020308794828));
#40327=DIRECTION('center_axis',(-1.,0.,0.));
#40328=DIRECTION('ref_axis',(0.,1.,0.));
#40329=DIRECTION('center_axis',(1.,0.,0.));
#40330=DIRECTION('ref_axis',(0.,0.,-1.));
#40331=DIRECTION('center_axis',(0.,-0.985836341420512,-0.167710190312393));
#40332=DIRECTION('ref_axis',(0.,0.167710190312393,-0.985836341420512));
#40333=DIRECTION('',(0.,-0.167710190312393,0.985836341420512));
#40334=DIRECTION('',(1.,0.,0.));
#40335=DIRECTION('center_axis',(1.,0.,0.));
#40336=DIRECTION('ref_axis',(0.,0.20791169081776,0.978147600733806));
#40337=DIRECTION('center_axis',(1.,0.,0.));
#40338=DIRECTION('ref_axis',(0.,0.20791169081776,0.978147600733806));
#40339=DIRECTION('',(-1.,0.,0.));
#40340=DIRECTION('center_axis',(-1.,0.,0.));
#40341=DIRECTION('ref_axis',(0.,0.20791169081776,0.978147600733806));
#40342=DIRECTION('center_axis',(0.,-0.832392431866445,0.554186646691768));
#40343=DIRECTION('ref_axis',(1.,0.,0.));
#40344=DIRECTION('',(0.,0.554186646691768,0.832392431866445));
#40345=DIRECTION('center_axis',(-1.,0.,0.));
#40346=DIRECTION('ref_axis',(0.,-1.,1.01064309961486E-15));
#40347=DIRECTION('center_axis',(1.,0.,0.));
#40348=DIRECTION('ref_axis',(0.,0.,-1.));
#40349=DIRECTION('center_axis',(0.,-0.832392431866443,-0.55418664669177));
#40350=DIRECTION('ref_axis',(-1.,0.,0.));
#40351=DIRECTION('',(0.,-0.55418664669177,0.832392431866443));
#40352=DIRECTION('',(1.,0.,0.));
#40353=DIRECTION('center_axis',(1.,0.,0.));
#40354=DIRECTION('ref_axis',(0.,-0.207911690817759,0.978147600733806));
#40355=DIRECTION('center_axis',(1.,0.,0.));
#40356=DIRECTION('ref_axis',(0.,-0.207911690817759,0.978147600733806));
#40357=DIRECTION('',(-1.,0.,0.));
#40358=DIRECTION('center_axis',(-1.,0.,0.));
#40359=DIRECTION('ref_axis',(0.,-0.207911690817759,0.978147600733806));
#40360=DIRECTION('center_axis',(0.,-0.985836341420512,0.167710190312393));
#40361=DIRECTION('ref_axis',(0.,-0.167710190312393,-0.985836341420512));
#40362=DIRECTION('',(0.,0.167710190312393,0.985836341420512));
#40363=DIRECTION('center_axis',(-1.,0.,0.));
#40364=DIRECTION('ref_axis',(0.,1.,0.));
#40365=DIRECTION('center_axis',(1.,0.,0.));
#40366=DIRECTION('ref_axis',(0.,0.,-1.));
#40367=DIRECTION('center_axis',(0.,-0.535020308794824,-0.844839197230509));
#40368=DIRECTION('ref_axis',(-1.,0.,0.));
#40369=DIRECTION('',(0.,-0.844839197230509,0.535020308794824));
#40370=DIRECTION('',(1.,0.,0.));
#40371=DIRECTION('center_axis',(1.,0.,0.));
#40372=DIRECTION('ref_axis',(0.,-0.587785252292473,0.809016994374947));
#40373=DIRECTION('center_axis',(1.,0.,0.));
#40374=DIRECTION('ref_axis',(0.,-0.587785252292473,0.809016994374947));
#40375=DIRECTION('',(-1.,0.,0.));
#40376=DIRECTION('center_axis',(-1.,0.,0.));
#40377=DIRECTION('ref_axis',(0.,-0.587785252292473,0.809016994374947));
#40378=DIRECTION('center_axis',(0.,-0.968820191500975,-0.247764881571247));
#40379=DIRECTION('ref_axis',(0.,0.247764881571247,-0.968820191500975));
#40380=DIRECTION('',(0.,-0.247764881571247,0.968820191500975));
#40381=DIRECTION('center_axis',(-1.,0.,0.));
#40382=DIRECTION('ref_axis',(0.,1.,0.));
#40383=DIRECTION('center_axis',(1.,0.,0.));
#40384=DIRECTION('ref_axis',(0.,0.,-1.));
#40385=DIRECTION('center_axis',(0.,-0.145138313825664,-0.989411375444938));
#40386=DIRECTION('ref_axis',(-1.,0.,0.));
#40387=DIRECTION('',(0.,-0.989411375444938,0.145138313825664));
#40388=DIRECTION('',(1.,0.,0.));
#40389=DIRECTION('center_axis',(1.,0.,0.));
#40390=DIRECTION('ref_axis',(0.,-0.866025403784438,0.5));
#40391=DIRECTION('center_axis',(1.,0.,0.));
#40392=DIRECTION('ref_axis',(0.,-0.866025403784438,0.5));
#40393=DIRECTION('',(-1.,0.,0.));
#40394=DIRECTION('center_axis',(-1.,0.,0.));
#40395=DIRECTION('ref_axis',(0.,-0.866025403784438,0.5));
#40396=DIRECTION('center_axis',(0.,-0.784286229015789,-0.620399154557929));
#40397=DIRECTION('ref_axis',(-1.,0.,0.));
#40398=DIRECTION('',(0.,-0.620399154557929,0.784286229015789));
#40399=DIRECTION('center_axis',(-1.,0.,0.));
#40400=DIRECTION('ref_axis',(0.,1.,0.));
#40401=DIRECTION('center_axis',(1.,0.,0.));
#40402=DIRECTION('ref_axis',(0.,0.,-1.));
#40403=DIRECTION('center_axis',(0.,0.269839414144142,-0.962905338324773));
#40404=DIRECTION('ref_axis',(-1.,0.,0.));
#40405=DIRECTION('',(0.,-0.962905338324773,-0.269839414144142));
#40406=DIRECTION('',(1.,0.,0.));
#40407=DIRECTION('center_axis',(1.,0.,0.));
#40408=DIRECTION('ref_axis',(0.,-0.994521895368273,0.104528463267654));
#40409=DIRECTION('center_axis',(1.,0.,0.));
#40410=DIRECTION('ref_axis',(0.,-0.994521895368273,0.104528463267654));
#40411=DIRECTION('',(-1.,0.,0.));
#40412=DIRECTION('center_axis',(-1.,0.,0.));
#40413=DIRECTION('ref_axis',(0.,-0.994521895368273,0.104528463267654));
#40414=DIRECTION('center_axis',(0.,-0.464142052517059,-0.885760777572168));
#40415=DIRECTION('ref_axis',(-1.,0.,0.));
#40416=DIRECTION('',(0.,-0.885760777572168,0.46414205251706));
#40417=DIRECTION('center_axis',(-1.,0.,0.));
#40418=DIRECTION('ref_axis',(0.,1.,0.));
#40419=DIRECTION('center_axis',(1.,0.,0.));
#40420=DIRECTION('ref_axis',(0.,0.,-1.));
#40421=DIRECTION('center_axis',(0.,0.63815945599431,-0.769904220487877));
#40422=DIRECTION('ref_axis',(-1.,0.,0.));
#40423=DIRECTION('',(0.,-0.769904220487877,-0.63815945599431));
#40424=DIRECTION('',(1.,0.,0.));
#40425=DIRECTION('center_axis',(1.,0.,0.));
#40426=DIRECTION('ref_axis',(0.,-0.951056516295154,-0.309016994374947));
#40427=DIRECTION('center_axis',(1.,0.,0.));
#40428=DIRECTION('ref_axis',(0.,-0.951056516295154,-0.309016994374947));
#40429=DIRECTION('',(-1.,0.,0.));
#40430=DIRECTION('center_axis',(-1.,0.,0.));
#40431=DIRECTION('ref_axis',(0.,-0.951056516295154,-0.309016994374947));
#40432=DIRECTION('center_axis',(0.,-0.0637434985399613,-0.997966315260132));
#40433=DIRECTION('ref_axis',(-1.,0.,0.));
#40434=DIRECTION('',(0.,-0.997966315260132,0.0637434985399613));
#40435=DIRECTION('center_axis',(-1.,0.,0.));
#40436=DIRECTION('ref_axis',(0.,1.,0.));
#40437=DIRECTION('center_axis',(1.,0.,0.));
#40438=DIRECTION('ref_axis',(0.,0.,-1.));
#40439=DIRECTION('center_axis',(0.,0.896135930406403,-0.443779668568367));
#40440=DIRECTION('ref_axis',(0.,0.443779668568367,0.896135930406403));
#40441=DIRECTION('',(0.,-0.443779668568367,-0.896135930406403));
#40442=DIRECTION('',(1.,0.,0.));
#40443=DIRECTION('center_axis',(1.,0.,0.));
#40444=DIRECTION('ref_axis',(0.,-0.743144825477395,-0.669130606358858));
#40445=DIRECTION('center_axis',(1.,0.,0.));
#40446=DIRECTION('ref_axis',(0.,-0.743144825477395,-0.669130606358858));
#40447=DIRECTION('',(-1.,0.,0.));
#40448=DIRECTION('center_axis',(-1.,0.,0.));
#40449=DIRECTION('ref_axis',(0.,-0.743144825477395,-0.669130606358858));
#40450=DIRECTION('center_axis',(0.,0.347676885426203,-0.937614410800269));
#40451=DIRECTION('ref_axis',(-1.,0.,0.));
#40452=DIRECTION('',(0.,-0.937614410800269,-0.347676885426203));
#40453=DIRECTION('center_axis',(-1.,0.,0.));
#40454=DIRECTION('ref_axis',(0.,1.,0.));
#40455=DIRECTION('center_axis',(1.,0.,0.));
#40456=DIRECTION('ref_axis',(0.,0.,-1.));
#40457=DIRECTION('center_axis',(0.,0.999162361311885,-0.0409215803416567));
#40458=DIRECTION('ref_axis',(0.,0.0409215803416567,0.999162361311885));
#40459=DIRECTION('',(0.,-0.0409215803416567,-0.999162361311885));
#40460=DIRECTION('',(1.,0.,0.));
#40461=DIRECTION('center_axis',(1.,0.,0.));
#40462=DIRECTION('ref_axis',(0.,-0.406736643075801,-0.913545457642601));
#40463=DIRECTION('center_axis',(1.,0.,0.));
#40464=DIRECTION('ref_axis',(0.,-0.406736643075801,-0.913545457642601));
#40465=DIRECTION('',(-1.,0.,0.));
#40466=DIRECTION('center_axis',(-1.,0.,0.));
#40467=DIRECTION('ref_axis',(0.,-0.406736643075801,-0.913545457642601));
#40468=DIRECTION('center_axis',(0.,0.698980777356831,-0.715140456753525));
#40469=DIRECTION('ref_axis',(-1.,0.,0.));
#40470=DIRECTION('',(0.,-0.715140456753525,-0.698980777356831));
#40471=DIRECTION('center_axis',(0.707106781186543,0.353553390593276,0.612372435695799));
#40472=DIRECTION('ref_axis',(0.654653670707982,0.,-0.75592894601845));
#40473=DIRECTION('',(0.,0.866025403784439,-0.5));
#40474=DIRECTION('',(-0.654653670707982,3.1022589451942E-16,0.75592894601845));
#40475=DIRECTION('',(0.,-0.866025403784439,0.5));
#40476=DIRECTION('',(-0.654653670707982,0.654653670707973,0.377964473009225));
#40477=DIRECTION('center_axis',(0.707106781186543,-0.353553390593276,0.612372435695799));
#40478=DIRECTION('ref_axis',(0.654653670707982,0.,-0.75592894601845));
#40479=DIRECTION('',(0.,0.866025403784439,0.5));
#40480=DIRECTION('',(-0.654653670707982,-0.654653670707973,0.377964473009226));
#40481=DIRECTION('',(0.,-0.866025403784439,-0.5));
#40482=DIRECTION('center_axis',(0.707106781186543,-0.353553390593276,-0.612372435695799));
#40483=DIRECTION('ref_axis',(-0.654653670707982,0.,-0.75592894601845));
#40484=DIRECTION('',(0.,-0.866025403784439,0.5));
#40485=DIRECTION('',(-0.654653670707982,1.38861894618649E-16,-0.75592894601845));
#40486=DIRECTION('',(0.,0.866025403784439,-0.5));
#40487=DIRECTION('',(0.654653670707982,0.654653670707973,0.377964473009225));
#40488=DIRECTION('center_axis',(0.707106781186543,0.353553390593276,-0.612372435695799));
#40489=DIRECTION('ref_axis',(-0.654653670707982,0.,-0.75592894601845));
#40490=DIRECTION('',(0.,0.866025403784439,0.5));
#40491=DIRECTION('',(0.,-0.866025403784439,-0.5));
#40492=DIRECTION('',(-0.654653670707982,0.654653670707973,-0.377964473009225));
#40493=DIRECTION('center_axis',(0.707106781186542,-0.707106781186553,2.26623325918421E-16));
#40494=DIRECTION('ref_axis',(3.20493781063932E-16,0.,-1.));
#40495=DIRECTION('',(0.,3.20493781063927E-16,1.));
#40496=DIRECTION('',(0.,-3.20493781063927E-16,-1.));
#40497=DIRECTION('center_axis',(0.707106781186543,0.707106781186552,1.13311662959211E-16));
#40498=DIRECTION('ref_axis',(1.60246890531966E-16,0.,-1.));
#40499=DIRECTION('',(0.,-1.60246890531964E-16,1.));
#40500=DIRECTION('',(0.,1.60246890531964E-16,-1.));
#40501=DIRECTION('center_axis',(0.,0.5,-0.866025403784439));
#40502=DIRECTION('ref_axis',(0.,-0.866025403784439,-0.5));
#40503=DIRECTION('',(-1.,0.,0.));
#40504=DIRECTION('',(0.,-0.866025403784439,-0.5));
#40505=DIRECTION('',(-1.,0.,0.));
#40506=DIRECTION('center_axis',(0.,1.,-3.20493781063927E-16));
#40507=DIRECTION('ref_axis',(0.,-3.20493781063927E-16,-1.));
#40508=DIRECTION('',(-1.,0.,0.));
#40509=DIRECTION('',(0.,-3.20493781063927E-16,-1.));
#40510=DIRECTION('center_axis',(0.,0.5,0.866025403784439));
#40511=DIRECTION('ref_axis',(0.,0.866025403784439,-0.5));
#40512=DIRECTION('',(-1.,0.,0.));
#40513=DIRECTION('',(0.,0.866025403784439,-0.5));
#40514=DIRECTION('center_axis',(1.,0.,0.));
#40515=DIRECTION('ref_axis',(0.,0.,-1.));
#40516=DIRECTION('center_axis',(1.,0.,0.));
#40517=DIRECTION('ref_axis',(0.,0.,-1.));
#40518=DIRECTION('center_axis',(0.,-0.5,0.866025403784439));
#40519=DIRECTION('ref_axis',(0.,0.866025403784439,0.5));
#40520=DIRECTION('',(-1.,0.,0.));
#40521=DIRECTION('',(0.,0.866025403784439,0.5));
#40522=DIRECTION('center_axis',(0.,-1.,-1.60246890531964E-16));
#40523=DIRECTION('ref_axis',(0.,-1.60246890531964E-16,1.));
#40524=DIRECTION('',(-1.,0.,0.));
#40525=DIRECTION('',(0.,-1.60246890531964E-16,1.));
#40526=DIRECTION('center_axis',(0.,-0.5,-0.866025403784439));
#40527=DIRECTION('ref_axis',(0.,-0.866025403784439,0.5));
#40528=DIRECTION('',(0.,-0.866025403784439,0.5));
#40529=DIRECTION('center_axis',(-1.,0.,0.));
#40530=DIRECTION('ref_axis',(0.,0.,1.));
#40531=DIRECTION('center_axis',(1.,0.,0.));
#40532=DIRECTION('ref_axis',(0.,-0.406736643075801,-0.913545457642601));
#40533=DIRECTION('center_axis',(1.,0.,0.));
#40534=DIRECTION('ref_axis',(0.,-0.743144825477395,-0.669130606358858));
#40535=DIRECTION('center_axis',(1.,0.,0.));
#40536=DIRECTION('ref_axis',(0.,-0.951056516295154,-0.309016994374947));
#40537=DIRECTION('center_axis',(1.,0.,0.));
#40538=DIRECTION('ref_axis',(0.,-0.994521895368273,0.104528463267654));
#40539=DIRECTION('center_axis',(1.,0.,0.));
#40540=DIRECTION('ref_axis',(0.,-0.866025403784438,0.5));
#40541=DIRECTION('center_axis',(1.,0.,0.));
#40542=DIRECTION('ref_axis',(0.,-0.587785252292473,0.809016994374947));
#40543=DIRECTION('center_axis',(1.,0.,0.));
#40544=DIRECTION('ref_axis',(0.,-0.207911690817759,0.978147600733806));
#40545=DIRECTION('center_axis',(1.,0.,0.));
#40546=DIRECTION('ref_axis',(0.,0.20791169081776,0.978147600733805));
#40547=DIRECTION('center_axis',(1.,0.,0.));
#40548=DIRECTION('ref_axis',(0.,0.587785252292473,0.809016994374947));
#40549=DIRECTION('center_axis',(1.,0.,0.));
#40550=DIRECTION('ref_axis',(0.,0.866025403784439,0.5));
#40551=DIRECTION('center_axis',(1.,0.,0.));
#40552=DIRECTION('ref_axis',(0.,0.994521895368273,0.104528463267653));
#40553=DIRECTION('center_axis',(1.,0.,0.));
#40554=DIRECTION('ref_axis',(0.,0.951056516295154,-0.309016994374948));
#40555=DIRECTION('center_axis',(1.,0.,0.));
#40556=DIRECTION('ref_axis',(0.,0.743144825477394,-0.669130606358858));
#40557=DIRECTION('center_axis',(1.,0.,0.));
#40558=DIRECTION('ref_axis',(0.,0.4067366430758,-0.913545457642601));
#40559=DIRECTION('center_axis',(1.,0.,0.));
#40560=DIRECTION('ref_axis',(0.,0.,-1.));
#40561=DIRECTION('center_axis',(-1.,0.,0.));
#40562=DIRECTION('ref_axis',(0.,1.,0.));
#40563=DIRECTION('center_axis',(1.,0.,0.));
#40564=DIRECTION('ref_axis',(0.,1.,0.));
#40565=DIRECTION('center_axis',(1.,0.,0.));
#40566=DIRECTION('ref_axis',(0.,0.,-1.));
#40567=DIRECTION('',(-0.707106781186544,0.707106781186551,8.65956056235498E-17));
#40568=DIRECTION('center_axis',(1.,0.,0.));
#40569=DIRECTION('ref_axis',(0.,1.,0.));
#40570=DIRECTION('center_axis',(1.,0.,0.));
#40571=DIRECTION('ref_axis',(0.,0.,-1.));
#40572=DIRECTION('',(-1.,0.,0.));
#40573=DIRECTION('center_axis',(-1.,0.,0.));
#40574=DIRECTION('ref_axis',(0.,0.,1.));
#40575=DIRECTION('center_axis',(1.,0.,0.));
#40576=DIRECTION('ref_axis',(0.,0.,-1.));
#40577=DIRECTION('center_axis',(1.,0.,0.));
#40578=DIRECTION('ref_axis',(0.,1.,0.));
#40579=DIRECTION('',(-0.70710678118655,0.707106781186545,8.6595605623549E-17));
#40580=DIRECTION('center_axis',(-1.,0.,0.));
#40581=DIRECTION('ref_axis',(0.,0.,1.));
#80263=CARTESIAN_POINT('',(0.,0.,0.));
#80264=CARTESIAN_POINT('Origin',(27.25,0.,0.));
#80265=CARTESIAN_POINT('',(27.,5.55,-6.79678973526781E-16));
#80266=CARTESIAN_POINT('Origin',(27.,0.,0.));
#80267=CARTESIAN_POINT('',(27.5,5.05,6.18446633569413E-16));
#80268=CARTESIAN_POINT('',(27.25,5.3,-6.49062803548097E-16));
#80269=CARTESIAN_POINT('',(27.5,-5.05,-6.18446633569413E-16));
#80270=CARTESIAN_POINT('Origin',(27.5,0.,0.));
#80271=CARTESIAN_POINT('Origin',(27.5,0.,0.));
#80272=CARTESIAN_POINT('Origin',(38.,0.,0.));
#80273=CARTESIAN_POINT('',(49.,-5.05,-6.18446633569413E-16));
#80274=CARTESIAN_POINT('Origin',(49.,0.,0.));
#80275=CARTESIAN_POINT('',(38.,-5.05,-6.18446633569413E-16));
#80276=CARTESIAN_POINT('Origin',(27.,7.6,0.));
#80277=CARTESIAN_POINT('',(27.,-7.6,-9.30731567351989E-16));
#80278=CARTESIAN_POINT('Origin',(27.,0.,0.));
#80279=CARTESIAN_POINT('Origin',(41.725,9.16562810019684,-1.42563428843676));
#80280=CARTESIAN_POINT('',(54.3836840636427,9.00782597316669,-1.02818086692503));
#80281=CARTESIAN_POINT('',(53.95,9.32343022722099,-1.82308770994211));
#80282=CARTESIAN_POINT('Ctrl Pts',(54.3836840636427,9.00782597316669,-1.02818086692503));
#80283=CARTESIAN_POINT('Ctrl Pts',(54.1865412262364,9.16194205564155,-1.41635031333084));
#80284=CARTESIAN_POINT('Ctrl Pts',(53.95,9.32343022722099,-1.82308770994211));
#80285=CARTESIAN_POINT('',(30.5,9.32343022722099,-1.82308770994211));
#80286=CARTESIAN_POINT('',(41.725,9.32343022722099,-1.82308770994211));
#80287=CARTESIAN_POINT('',(30.5,9.00782597317269,-1.0281808669314));
#80288=CARTESIAN_POINT('',(30.5,8.98477062633365,-0.970111773326804));
#80289=CARTESIAN_POINT('',(41.725,9.00782597317269,-1.02818086693141));
#80290=CARTESIAN_POINT('Origin',(30.5,10.1,0.));
#80291=CARTESIAN_POINT('',(30.5,9.00782597317269,1.0281808669314));
#80292=CARTESIAN_POINT('Origin',(30.5,10.1,0.));
#80293=CARTESIAN_POINT('',(54.3836840636427,9.00782597316669,1.02818086692503));
#80294=CARTESIAN_POINT('',(41.725,9.00782597317269,1.02818086693141));
#80295=CARTESIAN_POINT('',(54.75,8.68564356435644,0.499595709502806));
#80296=CARTESIAN_POINT('Ctrl Pts',(54.75,8.68564356435643,0.499595709502812));
#80297=CARTESIAN_POINT('Ctrl Pts',(54.687196533521,8.73974159983834,0.652747354291056));
#80298=CARTESIAN_POINT('Ctrl Pts',(54.5981025051697,8.81720407288878,0.789394637203874));
#80299=CARTESIAN_POINT('Ctrl Pts',(54.4672398095032,8.93309472235716,0.944212036355286));
#80300=CARTESIAN_POINT('Ctrl Pts',(54.4264645321808,8.9694238698269,0.987388647197093));
#80301=CARTESIAN_POINT('Ctrl Pts',(54.3836840636385,9.00782597316448,1.02818086692269));
#80302=CARTESIAN_POINT('',(54.75,8.68564356435644,-0.499595709502806));
#80303=CARTESIAN_POINT('Origin',(54.75,10.1,0.));
#80304=CARTESIAN_POINT('Ctrl Pts',(54.3836840636385,9.00782597316448,-1.02818086692269));
#80305=CARTESIAN_POINT('Ctrl Pts',(54.4264645321807,8.9694238698269,-0.987388647197093));
#80306=CARTESIAN_POINT('Ctrl Pts',(54.4672398095032,8.93309472235716,-0.944212036355286));
#80307=CARTESIAN_POINT('Ctrl Pts',(54.5981025051697,8.81720407288878,-0.789394637203873));
#80308=CARTESIAN_POINT('Ctrl Pts',(54.687196533521,8.73974159983834,-0.65274735429106));
#80309=CARTESIAN_POINT('Ctrl Pts',(54.75,8.68564356435643,-0.499595709502813));
#80310=CARTESIAN_POINT('Origin',(41.725,9.16562810019684,1.42563428843676));
#80311=CARTESIAN_POINT('',(53.95,9.32343022722099,1.82308770994211));
#80312=CARTESIAN_POINT('Ctrl Pts',(53.95,9.32343022722099,1.82308770994211));
#80313=CARTESIAN_POINT('Ctrl Pts',(54.1865412262364,9.16194205564153,1.41635031333086));
#80314=CARTESIAN_POINT('Ctrl Pts',(54.3836840636427,9.00782597316669,1.02818086692503));
#80315=CARTESIAN_POINT('',(30.5,9.32343022722099,1.82308770994211));
#80316=CARTESIAN_POINT('',(30.5,8.98477062633365,0.970111773326804));
#80317=CARTESIAN_POINT('',(41.725,9.32343022722099,1.82308770994211));
#80318=CARTESIAN_POINT('Origin',(54.35,0.,0.));
#80319=CARTESIAN_POINT('',(53.95,9.25889390890006,2.12670721626964));
#80320=CARTESIAN_POINT('Origin',(53.95,0.,0.));
#80321=CARTESIAN_POINT('',(54.3836840636427,8.64725733530933,2.72452293712243));
#80322=CARTESIAN_POINT('Ctrl Pts',(54.3836840636427,8.64725733530933,2.72452293712243));
#80323=CARTESIAN_POINT('Ctrl Pts',(54.1865412262364,8.94593211997956,2.4325971605926));
#80324=CARTESIAN_POINT('Ctrl Pts',(53.95,9.25889390890006,2.12670721626964));
#80325=CARTESIAN_POINT('',(54.75,8.13793410669876,3.07636611524524));
#80326=CARTESIAN_POINT('Ctrl Pts',(54.3836840636385,8.64725733530636,2.72452293712367));
#80327=CARTESIAN_POINT('Ctrl Pts',(54.4264645321807,8.59558357772359,2.74616894156256));
#80328=CARTESIAN_POINT('Ctrl Pts',(54.4672398095032,8.5448337403194,2.77083634278586));
#80329=CARTESIAN_POINT('Ctrl Pts',(54.5981025051697,8.37599245469372,2.86513210081603));
#80330=CARTESIAN_POINT('Ctrl Pts',(54.687196533521,8.24964750716334,2.95845877916735));
#80331=CARTESIAN_POINT('Ctrl Pts',(54.75,8.13793410669875,3.07636611524524));
#80332=CARTESIAN_POINT('Origin',(54.75,0.,0.));
#80333=CARTESIAN_POINT('Origin',(41.725,0.,0.));
#80334=CARTESIAN_POINT('',(53.95,9.25889390890006,-2.12670721626965));
#80335=CARTESIAN_POINT('Origin',(53.95,0.,0.));
#80336=CARTESIAN_POINT('',(30.5,9.25889390890006,-2.12670721626965));
#80337=CARTESIAN_POINT('',(41.725,9.25889390890006,-2.12670721626965));
#80338=CARTESIAN_POINT('',(30.5,7.77586075855085,-5.45765420887298));
#80339=CARTESIAN_POINT('Origin',(30.5,0.,0.));
#80340=CARTESIAN_POINT('',(53.95,7.77586075855085,-5.45765420887298));
#80341=CARTESIAN_POINT('',(41.725,7.77586075855085,-5.45765420887298));
#80342=CARTESIAN_POINT('',(53.95,7.59341071931979,-5.70877514425986));
#80343=CARTESIAN_POINT('Origin',(53.95,0.,0.));
#80344=CARTESIAN_POINT('',(30.5,7.59341071931979,-5.70877514425986));
#80345=CARTESIAN_POINT('',(41.725,7.59341071931979,-5.70877514425986));
#80346=CARTESIAN_POINT('',(30.5,4.88377432324997,-8.14854271385775));
#80347=CARTESIAN_POINT('Origin',(30.5,0.,0.));
#80348=CARTESIAN_POINT('',(53.95,4.88377432324997,-8.14854271385775));
#80349=CARTESIAN_POINT('',(41.725,4.88377432324997,-8.14854271385775));
#80350=CARTESIAN_POINT('',(53.95,4.61495783239841,-8.30374398721351));
#80351=CARTESIAN_POINT('Origin',(53.95,0.,0.));
#80352=CARTESIAN_POINT('',(30.5,4.61495783239841,-8.30374398721351));
#80353=CARTESIAN_POINT('',(41.725,4.61495783239841,-8.30374398721351));
#80354=CARTESIAN_POINT('',(30.5,1.14723893976231,-9.43047415642994));
#80355=CARTESIAN_POINT('Origin',(30.5,0.,0.));
#80356=CARTESIAN_POINT('',(53.95,1.14723893976231,-9.43047415642994));
#80357=CARTESIAN_POINT('',(41.725,1.14723893976231,-9.43047415642994));
#80358=CARTESIAN_POINT('',(53.95,0.838536810679625,-9.46292005763206));
#80359=CARTESIAN_POINT('Origin',(53.95,0.,0.));
#80360=CARTESIAN_POINT('',(30.5,0.838536810679625,-9.46292005763206));
#80361=CARTESIAN_POINT('',(41.725,0.838536810679625,-9.46292005763206));
#80362=CARTESIAN_POINT('',(30.5,-2.78766447874883,-9.08179094418727));
#80363=CARTESIAN_POINT('Origin',(30.5,0.,0.));
#80364=CARTESIAN_POINT('',(53.95,-2.78766447874883,-9.08179094418727));
#80365=CARTESIAN_POINT('',(41.725,-2.78766447874883,-9.08179094418727));
#80366=CARTESIAN_POINT('',(53.95,-3.08287484347344,-8.98587128215615));
#80367=CARTESIAN_POINT('Origin',(53.95,0.,0.));
#80368=CARTESIAN_POINT('',(30.5,-3.08287484347344,-8.98587128215615));
#80369=CARTESIAN_POINT('',(41.725,-3.08287484347344,-8.98587128215615));
#80370=CARTESIAN_POINT('',(30.5,-6.24055538374756,-7.16278357221404));
#80371=CARTESIAN_POINT('Origin',(30.5,0.,0.));
#80372=CARTESIAN_POINT('',(53.95,-6.24055538374756,-7.16278357221404));
#80373=CARTESIAN_POINT('',(41.725,-6.24055538374756,-7.16278357221404));
#80374=CARTESIAN_POINT('',(53.95,-6.47122943015123,-6.95508372791763));
#80375=CARTESIAN_POINT('Origin',(53.95,0.,0.));
#80376=CARTESIAN_POINT('',(30.5,-6.47122943015123,-6.95508372791763));
#80377=CARTESIAN_POINT('',(41.725,-6.47122943015123,-6.95508372791763));
#80378=CARTESIAN_POINT('',(30.5,-8.61439756923049,-4.00526584875909));
#80379=CARTESIAN_POINT('Origin',(30.5,0.,0.));
#80380=CARTESIAN_POINT('',(53.95,-8.61439756923049,-4.00526584875909));
#80381=CARTESIAN_POINT('',(41.725,-8.61439756923049,-4.00526584875909));
#80382=CARTESIAN_POINT('',(53.95,-8.74064965908211,-3.72169901217008));
#80383=CARTESIAN_POINT('Origin',(53.95,0.,0.));
#80384=CARTESIAN_POINT('',(30.5,-8.74064965908211,-3.72169901217008));
#80385=CARTESIAN_POINT('',(41.725,-8.74064965908211,-3.72169901217008));
#80386=CARTESIAN_POINT('',(30.5,-9.49873215564839,-0.155201273355761));
#80387=CARTESIAN_POINT('Origin',(30.5,0.,0.));
#80388=CARTESIAN_POINT('',(53.95,-9.49873215564839,-0.155201273355761));
#80389=CARTESIAN_POINT('',(41.725,-9.49873215564839,-0.155201273355761));
#80390=CARTESIAN_POINT('',(53.95,-9.5,-1.16341445918999E-15));
#80391=CARTESIAN_POINT('Origin',(53.95,0.,0.));
#80392=CARTESIAN_POINT('',(29.5,-9.5,-1.16341445918999E-15));
#80393=CARTESIAN_POINT('',(41.725,-9.5,-1.16341445918999E-15));
#80394=CARTESIAN_POINT('Origin',(29.5,0.,0.));
#80395=CARTESIAN_POINT('',(53.95,-9.49873215564839,0.155201273355763));
#80396=CARTESIAN_POINT('Origin',(53.95,0.,0.));
#80397=CARTESIAN_POINT('',(30.5,-9.49873215564839,0.155201273355763));
#80398=CARTESIAN_POINT('',(41.725,-9.49873215564839,0.155201273355763));
#80399=CARTESIAN_POINT('',(30.5,-8.74064965908211,3.72169901217009));
#80400=CARTESIAN_POINT('Origin',(30.5,0.,0.));
#80401=CARTESIAN_POINT('',(53.95,-8.74064965908211,3.72169901217008));
#80402=CARTESIAN_POINT('',(41.725,-8.74064965908211,3.72169901217009));
#80403=CARTESIAN_POINT('',(53.95,-8.61439756923049,4.00526584875909));
#80404=CARTESIAN_POINT('Origin',(53.95,0.,0.));
#80405=CARTESIAN_POINT('',(30.5,-8.61439756923049,4.00526584875909));
#80406=CARTESIAN_POINT('',(41.725,-8.61439756923049,4.00526584875909));
#80407=CARTESIAN_POINT('',(30.5,-6.47122943015123,6.95508372791763));
#80408=CARTESIAN_POINT('Origin',(30.5,0.,0.));
#80409=CARTESIAN_POINT('',(53.95,-6.47122943015123,6.95508372791763));
#80410=CARTESIAN_POINT('',(41.725,-6.47122943015123,6.95508372791763));
#80411=CARTESIAN_POINT('',(53.95,-6.24055538374755,7.16278357221405));
#80412=CARTESIAN_POINT('Origin',(53.95,0.,0.));
#80413=CARTESIAN_POINT('',(30.5,-6.24055538374755,7.16278357221405));
#80414=CARTESIAN_POINT('',(41.725,-6.24055538374755,7.16278357221405));
#80415=CARTESIAN_POINT('',(30.5,-3.08287484347343,8.98587128215615));
#80416=CARTESIAN_POINT('Origin',(30.5,0.,0.));
#80417=CARTESIAN_POINT('',(53.95,-3.08287484347343,8.98587128215615));
#80418=CARTESIAN_POINT('',(41.725,-3.08287484347343,8.98587128215615));
#80419=CARTESIAN_POINT('',(53.95,-2.78766447874883,9.08179094418728));
#80420=CARTESIAN_POINT('Origin',(53.95,0.,0.));
#80421=CARTESIAN_POINT('',(30.5,-2.78766447874883,9.08179094418727));
#80422=CARTESIAN_POINT('',(41.725,-2.78766447874883,9.08179094418727));
#80423=CARTESIAN_POINT('',(30.5,0.83853681067963,9.46292005763206));
#80424=CARTESIAN_POINT('Origin',(30.5,0.,0.));
#80425=CARTESIAN_POINT('',(53.95,0.83853681067963,9.46292005763206));
#80426=CARTESIAN_POINT('',(41.725,0.83853681067963,9.46292005763206));
#80427=CARTESIAN_POINT('',(53.95,1.14723893976232,9.43047415642994));
#80428=CARTESIAN_POINT('Origin',(53.95,0.,0.));
#80429=CARTESIAN_POINT('',(30.5,1.14723893976232,9.43047415642994));
#80430=CARTESIAN_POINT('',(41.725,1.14723893976232,9.43047415642994));
#80431=CARTESIAN_POINT('',(30.5,4.61495783239842,8.30374398721351));
#80432=CARTESIAN_POINT('Origin',(30.5,0.,0.));
#80433=CARTESIAN_POINT('',(53.95,4.61495783239842,8.30374398721351));
#80434=CARTESIAN_POINT('',(41.725,4.61495783239842,8.30374398721351));
#80435=CARTESIAN_POINT('',(53.95,4.88377432324998,8.14854271385775));
#80436=CARTESIAN_POINT('Origin',(53.95,0.,0.));
#80437=CARTESIAN_POINT('',(30.5,4.88377432324998,8.14854271385775));
#80438=CARTESIAN_POINT('',(41.725,4.88377432324998,8.14854271385775));
#80439=CARTESIAN_POINT('',(30.5,7.5934107193198,5.70877514425986));
#80440=CARTESIAN_POINT('Origin',(30.5,0.,0.));
#80441=CARTESIAN_POINT('',(53.95,7.5934107193198,5.70877514425986));
#80442=CARTESIAN_POINT('',(41.725,7.5934107193198,5.70877514425986));
#80443=CARTESIAN_POINT('',(53.95,7.77586075855086,5.45765420887297));
#80444=CARTESIAN_POINT('Origin',(53.95,0.,0.));
#80445=CARTESIAN_POINT('',(30.5,7.77586075855086,5.45765420887297));
#80446=CARTESIAN_POINT('',(41.725,7.77586075855086,5.45765420887297));
#80447=CARTESIAN_POINT('',(30.5,9.25889390890006,2.12670721626964));
#80448=CARTESIAN_POINT('Origin',(30.5,0.,0.));
#80449=CARTESIAN_POINT('',(41.725,9.25889390890006,2.12670721626964));
#80450=CARTESIAN_POINT('Origin',(30.5,0.,0.));
#80451=CARTESIAN_POINT('Origin',(41.725,8.95307562210873,2.42561507669434));
#80452=CARTESIAN_POINT('',(30.5,8.6472573353174,2.72452293711905));
#80453=CARTESIAN_POINT('',(30.5,8.60257639973902,2.76819423943269));
#80454=CARTESIAN_POINT('',(41.725,8.6472573353174,2.72452293711904));
#80455=CARTESIAN_POINT('Origin',(30.5,9.22680912219027,4.10804009506558));
#80456=CARTESIAN_POINT('',(30.5,7.81085966673651,4.60310285835948));
#80457=CARTESIAN_POINT('Origin',(30.5,9.22680912219027,4.10804009506558));
#80458=CARTESIAN_POINT('',(54.3836840636427,7.81085966673362,4.60310285835122));
#80459=CARTESIAN_POINT('',(41.725,7.81085966673651,4.60310285835948));
#80460=CARTESIAN_POINT('',(54.75,7.73152634314227,3.98917289739329));
#80461=CARTESIAN_POINT('Ctrl Pts',(54.75,7.73152634314226,3.98917289739329));
#80462=CARTESIAN_POINT('Ctrl Pts',(54.687196533521,7.71865497184144,4.15108754016898));
#80463=CARTESIAN_POINT('Ctrl Pts',(54.5981025051697,7.73384100509704,4.30742787102608));
#80464=CARTESIAN_POINT('Ctrl Pts',(54.4672398095032,7.77674247228157,4.49599757651354));
#80465=CARTESIAN_POINT('Ctrl Pts',(54.4264645321808,7.79236929017938,4.55021776871212));
#80466=CARTESIAN_POINT('Ctrl Pts',(54.3836840636385,7.81085966673255,4.60310285834817));
#80467=CARTESIAN_POINT('Origin',(54.75,9.22680912219027,4.10804009506558));
#80468=CARTESIAN_POINT('Origin',(41.725,7.79336021264368,5.03037853361623));
#80469=CARTESIAN_POINT('Ctrl Pts',(53.95,7.77586075855086,5.45765420887297));
#80470=CARTESIAN_POINT('Ctrl Pts',(54.1865412262364,7.79376897625248,5.02039795094072));
#80471=CARTESIAN_POINT('Ctrl Pts',(54.3836840636427,7.81085966673362,4.60310285835122));
#80472=CARTESIAN_POINT('',(30.5,7.81341638755651,4.54067664728931));
#80473=CARTESIAN_POINT('Origin',(54.35,0.,0.));
#80474=CARTESIAN_POINT('',(54.3836840636427,6.7914993463103,6.00613197382757));
#80475=CARTESIAN_POINT('Ctrl Pts',(54.3836840636427,6.7914993463103,6.00613197382757));
#80476=CARTESIAN_POINT('Ctrl Pts',(54.1865412262364,7.18308924953125,5.86092648599811));
#80477=CARTESIAN_POINT('Ctrl Pts',(53.95,7.5934107193198,5.70877514425986));
#80478=CARTESIAN_POINT('',(54.75,6.18310191118245,6.12039629075862));
#80479=CARTESIAN_POINT('Ctrl Pts',(54.3836840636385,6.79149934630708,6.0061319738275));
#80480=CARTESIAN_POINT('Ctrl Pts',(54.4264645321807,6.73548879660653,6.00488897216444));
#80481=CARTESIAN_POINT('Ctrl Pts',(54.4672398095032,6.67909337720287,6.0067819460014));
#80482=CARTESIAN_POINT('Ctrl Pts',(54.5981025051697,6.48649564757953,6.02425146969684));
#80483=CARTESIAN_POINT('Ctrl Pts',(54.687196533521,6.33311441480502,6.05812051295347));
#80484=CARTESIAN_POINT('Ctrl Pts',(54.75,6.18310191118246,6.12039629075861));
#80485=CARTESIAN_POINT('Origin',(54.75,0.,0.));
#80486=CARTESIAN_POINT('Origin',(41.725,7.19245503281942,5.85745355904381));
#80487=CARTESIAN_POINT('',(30.5,6.79149934631905,6.00613197382777));
#80488=CARTESIAN_POINT('',(30.5,6.7329185616764,6.0278543199391));
#80489=CARTESIAN_POINT('',(41.725,6.79149934631905,6.00613197382777));
#80490=CARTESIAN_POINT('Origin',(30.5,6.75821912422447,7.50576273732168));
#80491=CARTESIAN_POINT('',(30.5,5.26332476448918,7.38210654770054));
#80492=CARTESIAN_POINT('Origin',(30.5,6.75821912422447,7.50576273732168));
#80493=CARTESIAN_POINT('',(54.3836840636427,5.2633247644899,7.38210654769182));
#80494=CARTESIAN_POINT('',(41.725,5.26332476448918,7.38210654770054));
#80495=CARTESIAN_POINT('',(54.75,5.44055797848702,6.78898585082641));
#80496=CARTESIAN_POINT('Ctrl Pts',(54.75,5.44055797848701,6.78898585082641));
#80497=CARTESIAN_POINT('Ctrl Pts',(54.687196533521,5.3629427774341,6.9316669789053));
#80498=CARTESIAN_POINT('Ctrl Pts',(54.5981025051697,5.3132265677842,7.08066769419416));
#80499=CARTESIAN_POINT('Ctrl Pts',(54.4672398095032,5.27572079926106,7.27038429083689));
#80500=CARTESIAN_POINT('Ctrl Pts',(54.4264645321808,5.26794326880725,7.32627290058613));
#80501=CARTESIAN_POINT('Ctrl Pts',(54.3836840636385,5.26332476449017,7.38210654768861));
#80502=CARTESIAN_POINT('Origin',(54.75,6.75821912422447,7.50576273732168));
#80503=CARTESIAN_POINT('Origin',(41.725,5.07354954386958,7.76532463077915));
#80504=CARTESIAN_POINT('Ctrl Pts',(53.95,4.88377432324998,8.14854271385775));
#80505=CARTESIAN_POINT('Ctrl Pts',(54.1865412262364,5.07798243670107,7.75637317394928));
#80506=CARTESIAN_POINT('Ctrl Pts',(54.3836840636427,5.2633247644899,7.38210654769182));
#80507=CARTESIAN_POINT('',(30.5,5.29105147271138,7.32611727818317));
#80508=CARTESIAN_POINT('Origin',(54.35,0.,0.));
#80509=CARTESIAN_POINT('',(54.3836840636427,3.76142942149961,8.24922622826191));
#80510=CARTESIAN_POINT('Ctrl Pts',(54.3836840636427,3.76142942149961,8.24922622826192));
#80511=CARTESIAN_POINT('Ctrl Pts',(54.1865412262364,4.1782249915217,8.27584837712899));
#80512=CARTESIAN_POINT('Ctrl Pts',(53.95,4.61495783239842,8.30374398721351));
#80513=CARTESIAN_POINT('',(54.75,3.15915522350528,8.10615434554508));
#80514=CARTESIAN_POINT('Ctrl Pts',(54.3836840636385,3.76142942149669,8.24922622826054));
#80515=CARTESIAN_POINT('Ctrl Pts',(54.4264645321808,3.71076681256147,8.22530914677537));
#80516=CARTESIAN_POINT('Ctrl Pts',(54.4672398095032,3.65847709150953,8.20410038085247));
#80517=CARTESIAN_POINT('Ctrl Pts',(54.5981025051697,3.47542481503583,8.1417230308606));
#80518=CARTESIAN_POINT('Ctrl Pts',(54.687196533521,3.32152830558866,8.11027817375286));
#80519=CARTESIAN_POINT('Ctrl Pts',(54.75,3.15915522350528,8.10615434554507));
#80520=CARTESIAN_POINT('Origin',(54.75,0.,0.));
#80521=CARTESIAN_POINT('Origin',(41.725,4.18819362695297,8.27648510773958));
#80522=CARTESIAN_POINT('',(30.5,3.76142942150752,8.24922622826565));
#80523=CARTESIAN_POINT('',(30.5,3.69907793765504,8.2452436271907));
#80524=CARTESIAN_POINT('',(41.725,3.76142942150752,8.24922622826565));
#80525=CARTESIAN_POINT('Origin',(30.5,3.12107164318697,9.60567081458105));
#80526=CARTESIAN_POINT('',(30.5,1.8057131946573,8.88467695061159));
#80527=CARTESIAN_POINT('Origin',(30.5,3.12107164318697,9.60567081458105));
#80528=CARTESIAN_POINT('',(54.3836840636427,1.80571319466151,8.88467695060392));
#80529=CARTESIAN_POINT('',(41.725,1.8057131946573,8.88467695061159));
#80530=CARTESIAN_POINT('',(54.75,2.20886771343379,8.41492147465143));
#80531=CARTESIAN_POINT('Ctrl Pts',(54.75,2.20886771343378,8.41492147465143));
#80532=CARTESIAN_POINT('Ctrl Pts',(54.687196533521,2.07992905600282,8.51369822477129));
#80533=CARTESIAN_POINT('Ctrl Pts',(54.5981025051697,1.97390698775344,8.62959574718948));
#80534=CARTESIAN_POINT('Ctrl Pts',(54.4672398095032,1.86247907162951,8.78765551190679));
#80535=CARTESIAN_POINT('Ctrl Pts',(54.4264645321807,1.83264199849617,8.83554889084895));
#80536=CARTESIAN_POINT('Ctrl Pts',(54.3836840636385,1.80571319466305,8.88467695060109));
#80537=CARTESIAN_POINT('Origin',(54.75,3.12107164318697,9.60567081458105));
#80538=CARTESIAN_POINT('Origin',(41.725,1.47647606720981,9.15757555352076));
#80539=CARTESIAN_POINT('Ctrl Pts',(53.95,1.14723893976232,9.43047415642994));
#80540=CARTESIAN_POINT('Ctrl Pts',(54.1865412262364,1.48416660182181,9.15120101074399));
#80541=CARTESIAN_POINT('Ctrl Pts',(54.3836840636427,1.80571319466151,8.88467695060392));
#80542=CARTESIAN_POINT('',(30.5,1.85381569054083,8.8448056759931));
#80543=CARTESIAN_POINT('Origin',(54.35,0.,0.));
#80544=CARTESIAN_POINT('',(54.3836840636427,0.0809741781981114,9.06595432596218));
#80545=CARTESIAN_POINT('Ctrl Pts',(54.3836840636427,0.0809741781981114,
9.06595432596218));
#80546=CARTESIAN_POINT('Ctrl Pts',(54.1865412262363,0.450907674495694,9.25980090013203));
#80547=CARTESIAN_POINT('Ctrl Pts',(53.95,0.83853681067963,9.46292005763206));
#80548=CARTESIAN_POINT('',(54.75,-0.411038102340174,8.69028467188645));
#80549=CARTESIAN_POINT('Ctrl Pts',(54.3836840636385,0.0809741781960095,
9.06595432595974));
#80550=CARTESIAN_POINT('Ctrl Pts',(54.4264645321807,0.0444195353663552,
9.02349864532112));
#80551=CARTESIAN_POINT('Ctrl Pts',(54.4672398095032,0.005276880473219,8.98285532794201));
#80552=CARTESIAN_POINT('Ctrl Pts',(54.5981025051697,-0.136578541270811,
8.85141671475685));
#80553=CARTESIAN_POINT('Ctrl Pts',(54.687196533521,-0.264380222801317,8.76009505874624));
#80554=CARTESIAN_POINT('Ctrl Pts',(54.75,-0.411038102340168,8.69028467188645));
#80555=CARTESIAN_POINT('Origin',(54.75,0.,0.));
#80556=CARTESIAN_POINT('Origin',(41.725,0.459755494441725,9.26443719180043));
#80557=CARTESIAN_POINT('',(30.5,0.0809741782038195,9.06595432596881));
#80558=CARTESIAN_POINT('',(30.5,0.0256331331450422,9.03695540561423));
#80559=CARTESIAN_POINT('',(41.725,0.0809741782038194,9.06595432596881));
#80560=CARTESIAN_POINT('Origin',(30.5,-1.0557374790033,10.0446711432196));
#80561=CARTESIAN_POINT('',(30.5,-1.96412259092021,8.85100599400572));
#80562=CARTESIAN_POINT('Origin',(30.5,-1.0557374790033,10.0446711432196));
#80563=CARTESIAN_POINT('',(54.3836840636427,-1.96412259091325,8.85100599400042));
#80564=CARTESIAN_POINT('',(41.725,-1.96412259092021,8.85100599400572));
#80565=CARTESIAN_POINT('',(54.75,-1.40475584620535,8.58584072834757));
#80566=CARTESIAN_POINT('Ctrl Pts',(54.75,-1.40475584620535,8.58584072834756));
#80567=CARTESIAN_POINT('Ctrl Pts',(54.687196533521,-1.56272329477365,8.6236337030541));
#80568=CARTESIAN_POINT('Ctrl Pts',(54.5981025051697,-1.70671904284191,8.68638829807956));
#80569=CARTESIAN_POINT('Ctrl Pts',(54.4672398095032,-1.87280220757798,8.78546126162393));
#80570=CARTESIAN_POINT('Ctrl Pts',(54.4264645321808,-1.91953972238478,8.81707820944224));
#80571=CARTESIAN_POINT('Ctrl Pts',(54.3836840636385,-1.96412259091068,8.85100599399847));
#80572=CARTESIAN_POINT('Origin',(54.75,-1.0557374790033,10.0446711432196));
#80573=CARTESIAN_POINT('Origin',(41.725,-2.37589353483452,8.9663984690965));
#80574=CARTESIAN_POINT('Ctrl Pts',(53.95,-2.78766447874883,9.08179094418728));
#80575=CARTESIAN_POINT('Ctrl Pts',(54.1865412262364,-2.36627512174276,8.96370305672978));
#80576=CARTESIAN_POINT('Ctrl Pts',(54.3836840636427,-1.96412259091325,8.85100599400042));
#80577=CARTESIAN_POINT('',(30.5,-1.90396166591106,8.83414681988681));
#80578=CARTESIAN_POINT('Origin',(54.35,0.,0.));
#80579=CARTESIAN_POINT('',(54.3836840636427,-3.61348223614116,8.31509655909415));
#80580=CARTESIAN_POINT('Ctrl Pts',(54.3836840636427,-3.61348223614116,8.31509655909415));
#80581=CARTESIAN_POINT('Ctrl Pts',(54.1865412262364,-3.35437567581821,8.64264972485202));
#80582=CARTESIAN_POINT('Ctrl Pts',(53.95,-3.08287484347343,8.98587128215615));
#80583=CARTESIAN_POINT('',(54.75,-3.91015920612708,7.7717858297009));
#80584=CARTESIAN_POINT('Ctrl Pts',(54.3836840636385,-3.61348223614209,8.31509655909106));
#80585=CARTESIAN_POINT('Ctrl Pts',(54.4264645321808,-3.62960828303242,8.26144325217917));
#80586=CARTESIAN_POINT('Ctrl Pts',(54.4672398095032,-3.64883575113587,8.20839298215165));
#80587=CARTESIAN_POINT('Ctrl Pts',(54.5981025051697,-3.72496622701463,8.03062003607524));
#80588=CARTESIAN_POINT('Ctrl Pts',(54.687196533521,-3.80457500885003,7.89521192511718));
#80589=CARTESIAN_POINT('Ctrl Pts',(54.75,-3.91015920612707,7.77178582970089));
#80590=CARTESIAN_POINT('Origin',(54.75,0.,0.));
#80591=CARTESIAN_POINT('Origin',(41.725,-3.34817853980604,8.65048392062934));
#80592=CARTESIAN_POINT('',(30.5,-3.61348223613864,8.31509655910254));
#80593=CARTESIAN_POINT('',(30.5,-3.65224387295544,8.26609549624456));
#80594=CARTESIAN_POINT('',(41.725,-3.61348223613864,8.31509655910254));
#80595=CARTESIAN_POINT('Origin',(30.5,-5.05,8.74685657822283));
#80596=CARTESIAN_POINT('',(30.5,-5.39434373703405,7.28691569217113));
#80597=CARTESIAN_POINT('Origin',(30.5,-5.05,8.74685657822283));
#80598=CARTESIAN_POINT('',(54.3836840636427,-5.39434373702553,7.28691569216912));
#80599=CARTESIAN_POINT('',(41.725,-5.39434373703405,7.28691569217113));
#80600=CARTESIAN_POINT('',(54.75,-4.77548435822936,7.27219012019809));
#80601=CARTESIAN_POINT('Ctrl Pts',(54.75,-4.77548435822936,7.27219012019809));
#80602=CARTESIAN_POINT('Ctrl Pts',(54.687196533521,-4.9351665909883,7.24246457082613));
#80603=CARTESIAN_POINT('Ctrl Pts',(54.5981025051697,-5.09223784587414,7.24122539887136));
#80604=CARTESIAN_POINT('Ctrl Pts',(54.4672398095032,-5.2842589712213,7.26418094579636));
#80605=CARTESIAN_POINT('Ctrl Pts',(54.4264645321807,-5.33981558679448,7.27405460498208));
#80606=CARTESIAN_POINT('Ctrl Pts',(54.3836840636385,-5.3943437370224,7.28691569216838));
#80607=CARTESIAN_POINT('Origin',(54.75,-5.05,8.74685657822283));
#80608=CARTESIAN_POINT('Origin',(41.725,-5.8174495603908,7.22484963219259));
#80609=CARTESIAN_POINT('Ctrl Pts',(53.95,-6.24055538374755,7.16278357221405));
#80610=CARTESIAN_POINT('Ctrl Pts',(54.1865412262364,-5.8075663798233,7.22629941152117));
#80611=CARTESIAN_POINT('Ctrl Pts',(54.3836840636427,-5.39434373702553,7.28691569216912));
#80612=CARTESIAN_POINT('',(30.5,-5.3325267533782,7.29598372291776));
#80613=CARTESIAN_POINT('Origin',(54.35,0.,0.));
#80614=CARTESIAN_POINT('',(54.3836840636427,-6.68313474439608,6.126483056878));
#80615=CARTESIAN_POINT('Ctrl Pts',(54.3836840636427,-6.68313474439608,6.126483056878));
#80616=CARTESIAN_POINT('Ctrl Pts',(54.1865412262364,-6.57965699823688,6.53110589613716));
#80617=CARTESIAN_POINT('Ctrl Pts',(53.95,-6.47122943015123,6.95508372791763));
#80618=CARTESIAN_POINT('',(54.75,-6.73317826049339,5.50947461310234));
#80619=CARTESIAN_POINT('Ctrl Pts',(54.3836840636385,-6.68313474439567,6.1264830568748));
#80620=CARTESIAN_POINT('Ctrl Pts',(54.4264645321807,-6.6760438553388,6.07090926787968));
#80621=CARTESIAN_POINT('Ctrl Pts',(54.4672398095032,-6.67203153274142,6.01462491883807));
#80622=CARTESIAN_POINT('Ctrl Pts',(54.5981025051697,-6.66927341185182,5.82125619726353));
#80623=CARTESIAN_POINT('Ctrl Pts',(54.687196533521,-6.68692421238969,5.66517492388676));
#80624=CARTESIAN_POINT('Ctrl Pts',(54.75,-6.73317826049339,5.50947461310234));
#80625=CARTESIAN_POINT('Origin',(54.75,0.,0.));
#80626=CARTESIAN_POINT('Origin',(41.725,-6.57718208727421,6.54078339240215));
#80627=CARTESIAN_POINT('',(30.5,-6.68313474439718,6.12648305688668));
#80628=CARTESIAN_POINT('',(30.5,-6.69861473382796,6.06595258045413));
#80629=CARTESIAN_POINT('',(41.725,-6.68313474439718,6.12648305688668));
#80630=CARTESIAN_POINT('Origin',(30.5,-8.17107164318697,5.93663104815398));
#80631=CARTESIAN_POINT('',(30.5,-7.89183384494033,4.46285146760933));
#80632=CARTESIAN_POINT('Origin',(30.5,-8.17107164318697,5.93663104815398));
#80633=CARTESIAN_POINT('',(54.3836840636427,-7.89183384493173,4.46285146761096));
#80634=CARTESIAN_POINT('',(41.725,-7.89183384494033,4.46285146760933));
#80635=CARTESIAN_POINT('',(54.75,-7.32048824080211,4.70111177449315));
#80636=CARTESIAN_POINT('Ctrl Pts',(54.75,-7.32048824080211,4.70111177449315));
#80637=CARTESIAN_POINT('Ctrl Pts',(54.687196533521,-7.45427474904012,4.60900751857725));
#80638=CARTESIAN_POINT('Ctrl Pts',(54.5981025051697,-7.59726246382623,4.54398884373077));
#80639=CARTESIAN_POINT('Ctrl Pts',(54.4672398095032,-7.78201935275478,4.48685775142846));
#80640=CARTESIAN_POINT('Ctrl Pts',(54.4264645321807,-7.83678882554574,4.473280876609));
#80641=CARTESIAN_POINT('Ctrl Pts',(54.3836840636385,-7.89183384492856,4.46285146761156));
#80642=CARTESIAN_POINT('Origin',(54.75,-8.17107164318697,5.93663104815398));
#80643=CARTESIAN_POINT('Origin',(41.725,-8.25311570708541,4.23405865818421));
#80644=CARTESIAN_POINT('Ctrl Pts',(53.95,-8.61439756923049,4.00526584875909));
#80645=CARTESIAN_POINT('Ctrl Pts',(54.1865412262364,-8.2446766507482,4.23940294919136));
#80646=CARTESIAN_POINT('Ctrl Pts',(54.3836840636427,-7.89183384493173,4.46285146761096));
#80647=CARTESIAN_POINT('',(30.5,-7.83904952070155,4.49627875832492));
#80648=CARTESIAN_POINT('Origin',(54.35,0.,0.));
#80649=CARTESIAN_POINT('',(54.3836840636427,-8.5972125409718,2.87854497677634));
#80650=CARTESIAN_POINT('Ctrl Pts',(54.3836840636427,-8.5972125409718,2.87854497677635));
#80651=CARTESIAN_POINT('Ctrl Pts',(54.1865412262364,-8.66725585135303,3.29027452474581));
#80652=CARTESIAN_POINT('Ctrl Pts',(53.95,-8.74064965908211,3.72169901217008));
#80653=CARTESIAN_POINT('',(54.75,-8.39196962461624,2.29452518389281));
#80654=CARTESIAN_POINT('Ctrl Pts',(54.3836840636385,-8.59721254097013,2.87854497677359));
#80655=CARTESIAN_POINT('Ctrl Pts',(54.4264645321808,-8.5681307951027,2.83065991868452));
#80656=CARTESIAN_POINT('Ctrl Pts',(54.4672398095032,-8.54157244883238,2.78087356590539));
#80657=CARTESIAN_POINT('Ctrl Pts',(54.5981025051697,-8.46040263533297,2.60534427749265));
#80658=CARTESIAN_POINT('Ctrl Pts',(54.687196533521,-8.41304347080783,2.45557771181784));
#80659=CARTESIAN_POINT('Ctrl Pts',(54.75,-8.39196962461623,2.29452518389282));
#80660=CARTESIAN_POINT('Origin',(54.75,0.,0.));
#80661=CARTESIAN_POINT('Origin',(41.725,-8.66893110002923,3.30012199447695));
#80662=CARTESIAN_POINT('',(30.5,-8.59721254097634,2.87854497678382));
#80663=CARTESIAN_POINT('',(30.5,-8.58673425221723,2.816951356054));
#80664=CARTESIAN_POINT('',(41.725,-8.59721254097634,2.87854497678382));
#80665=CARTESIAN_POINT('Origin',(30.5,-9.87929076741144,2.09990807725937));
#80666=CARTESIAN_POINT('',(30.5,-9.0247541859967,0.867119680565108));
#80667=CARTESIAN_POINT('Origin',(30.5,-9.87929076741144,2.09990807725937));
#80668=CARTESIAN_POINT('',(54.3836840636427,-9.02475418598951,0.867119680570092));
#80669=CARTESIAN_POINT('',(41.725,-9.0247541859967,0.867119680565108));
#80670=CARTESIAN_POINT('',(54.75,-8.59971320199229,1.31716849471867));
#80671=CARTESIAN_POINT('Ctrl Pts',(54.75,-8.59971320199229,1.31716849471866));
#80672=CARTESIAN_POINT('Ctrl Pts',(54.687196533521,-8.68447108302277,1.17861119484757));
#80673=CARTESIAN_POINT('Ctrl Pts',(54.5981025051697,-8.78865138282002,1.06105533666644));
#80674=CARTESIAN_POINT('Ctrl Pts',(54.4672398095032,-8.93419789077059,0.93371609001558));
#80675=CARTESIAN_POINT('Ctrl Pts',(54.4264645321807,-8.97871008136871,0.899036246189251));
#80676=CARTESIAN_POINT('Ctrl Pts',(54.3836840636385,-9.02475418598686,0.867119680571931));
#80677=CARTESIAN_POINT('Origin',(54.75,-9.87929076741144,2.09990807725937));
#80678=CARTESIAN_POINT('Origin',(41.725,-9.26174317082255,0.511160476960435));
#80679=CARTESIAN_POINT('Ctrl Pts',(53.95,-9.49873215564839,0.155201273355763));
#80680=CARTESIAN_POINT('Ctrl Pts',(54.1865412262364,-9.2562074282228,0.519475203179616));
#80681=CARTESIAN_POINT('Ctrl Pts',(54.3836840636427,-9.02475418598951,0.867119680570092));
#80682=CARTESIAN_POINT('',(30.5,-8.99012941036642,0.919126349007539));
#80683=CARTESIAN_POINT('Origin',(54.35,0.,0.));
#80684=CARTESIAN_POINT('',(54.3836840636427,-9.02475418598951,-0.867119680570087));
#80685=CARTESIAN_POINT('Ctrl Pts',(54.3836840636427,-9.02475418598951,-0.867119680570087));
#80686=CARTESIAN_POINT('Ctrl Pts',(54.1865412262364,-9.25620742822278,-0.519475203179662));
#80687=CARTESIAN_POINT('Ctrl Pts',(53.95,-9.49873215564839,-0.155201273355761));
#80688=CARTESIAN_POINT('',(54.75,-8.59971320199229,-1.31716849471866));
#80689=CARTESIAN_POINT('Ctrl Pts',(54.3836840636385,-9.02475418598685,-0.867119680571927));
#80690=CARTESIAN_POINT('Ctrl Pts',(54.4264645321808,-8.97871008136871,-0.899036246189249));
#80691=CARTESIAN_POINT('Ctrl Pts',(54.4672398095032,-8.93419789077059,-0.933716090015573));
#80692=CARTESIAN_POINT('Ctrl Pts',(54.5981025051697,-8.78865138282002,-1.06105533666644));
#80693=CARTESIAN_POINT('Ctrl Pts',(54.687196533521,-8.68447108302277,-1.17861119484756));
#80694=CARTESIAN_POINT('Ctrl Pts',(54.75,-8.59971320199229,-1.31716849471866));
#80695=CARTESIAN_POINT('Origin',(54.75,0.,0.));
#80696=CARTESIAN_POINT('Origin',(41.725,-9.26174317082254,-0.511160476960432));
#80697=CARTESIAN_POINT('',(30.5,-9.0247541859967,-0.867119680565103));
#80698=CARTESIAN_POINT('',(30.5,-8.99012941036642,-0.919126349007532));
#80699=CARTESIAN_POINT('',(41.725,-9.0247541859967,-0.867119680565103));
#80700=CARTESIAN_POINT('Origin',(30.5,-9.87929076741144,-2.09990807725937));
#80701=CARTESIAN_POINT('',(30.5,-8.59721254097635,-2.87854497678382));
#80702=CARTESIAN_POINT('Origin',(30.5,-9.87929076741144,-2.09990807725937));
#80703=CARTESIAN_POINT('',(54.3836840636427,-8.5972125409718,-2.87854497677634));
#80704=CARTESIAN_POINT('',(41.725,-8.59721254097635,-2.87854497678382));
#80705=CARTESIAN_POINT('',(54.75,-8.39196962461624,-2.29452518389281));
#80706=CARTESIAN_POINT('Ctrl Pts',(54.75,-8.39196962461624,-2.29452518389281));
#80707=CARTESIAN_POINT('Ctrl Pts',(54.687196533521,-8.41304347080783,-2.45557771181783));
#80708=CARTESIAN_POINT('Ctrl Pts',(54.5981025051697,-8.46040263533297,-2.60534427749264));
#80709=CARTESIAN_POINT('Ctrl Pts',(54.4672398095032,-8.54157244883238,-2.78087356590538));
#80710=CARTESIAN_POINT('Ctrl Pts',(54.4264645321808,-8.5681307951027,-2.83065991868451));
#80711=CARTESIAN_POINT('Ctrl Pts',(54.3836840636385,-8.59721254097013,-2.87854497677358));
#80712=CARTESIAN_POINT('Origin',(54.75,-9.87929076741144,-2.09990807725937));
#80713=CARTESIAN_POINT('Origin',(41.725,-8.66893110002923,-3.30012199447695));
#80714=CARTESIAN_POINT('Ctrl Pts',(53.95,-8.74064965908211,-3.72169901217008));
#80715=CARTESIAN_POINT('Ctrl Pts',(54.1865412262364,-8.66725585135304,-3.29027452474592));
#80716=CARTESIAN_POINT('Ctrl Pts',(54.3836840636427,-8.5972125409718,-2.87854497677634));
#80717=CARTESIAN_POINT('',(30.5,-8.58673425221724,-2.816951356054));
#80718=CARTESIAN_POINT('Origin',(54.35,0.,0.));
#80719=CARTESIAN_POINT('',(54.3836840636427,-7.89183384493173,-4.46285146761096));
#80720=CARTESIAN_POINT('Ctrl Pts',(54.3836840636427,-7.89183384493173,-4.46285146761096));
#80721=CARTESIAN_POINT('Ctrl Pts',(54.1865412262364,-8.2446766507482,-4.23940294919137));
#80722=CARTESIAN_POINT('Ctrl Pts',(53.95,-8.61439756923049,-4.00526584875909));
#80723=CARTESIAN_POINT('',(54.75,-7.32048824080209,-4.70111177449316));
#80724=CARTESIAN_POINT('Ctrl Pts',(54.3836840636385,-7.89183384492855,-4.46285146761156));
#80725=CARTESIAN_POINT('Ctrl Pts',(54.4264645321808,-7.83678882554573,-4.473280876609));
#80726=CARTESIAN_POINT('Ctrl Pts',(54.4672398095032,-7.78201935275478,-4.48685775142846));
#80727=CARTESIAN_POINT('Ctrl Pts',(54.5981025051697,-7.59726246382623,-4.54398884373077));
#80728=CARTESIAN_POINT('Ctrl Pts',(54.687196533521,-7.45427474904011,-4.60900751857725));
#80729=CARTESIAN_POINT('Ctrl Pts',(54.75,-7.32048824080209,-4.70111177449316));
#80730=CARTESIAN_POINT('Origin',(54.75,0.,0.));
#80731=CARTESIAN_POINT('Origin',(41.725,-8.25311570708541,-4.23405865818421));
#80732=CARTESIAN_POINT('',(30.5,-7.89183384494032,-4.46285146760933));
#80733=CARTESIAN_POINT('',(30.5,-7.83904952070155,-4.49627875832492));
#80734=CARTESIAN_POINT('',(41.725,-7.89183384494032,-4.46285146760933));
#80735=CARTESIAN_POINT('Origin',(30.5,-8.17107164318697,-5.93663104815398));
#80736=CARTESIAN_POINT('',(30.5,-6.68313474439719,-6.12648305688667));
#80737=CARTESIAN_POINT('Origin',(30.5,-8.17107164318697,-5.93663104815398));
#80738=CARTESIAN_POINT('',(54.3836840636427,-6.68313474439608,-6.12648305687799));
#80739=CARTESIAN_POINT('',(41.725,-6.68313474439719,-6.12648305688667));
#80740=CARTESIAN_POINT('',(54.75,-6.73317826049341,-5.50947461310232));
#80741=CARTESIAN_POINT('Ctrl Pts',(54.75,-6.7331782604934,-5.50947461310232));
#80742=CARTESIAN_POINT('Ctrl Pts',(54.687196533521,-6.68692421238969,-5.66517492388675));
#80743=CARTESIAN_POINT('Ctrl Pts',(54.5981025051697,-6.66927341185182,-5.82125619726353));
#80744=CARTESIAN_POINT('Ctrl Pts',(54.4672398095033,-6.67203153274142,-6.01462491883807));
#80745=CARTESIAN_POINT('Ctrl Pts',(54.4264645321808,-6.6760438553388,-6.07090926787966));
#80746=CARTESIAN_POINT('Ctrl Pts',(54.3836840636385,-6.68313474439567,-6.12648305687479));
#80747=CARTESIAN_POINT('Origin',(54.75,-8.17107164318697,-5.93663104815398));
#80748=CARTESIAN_POINT('Origin',(41.725,-6.57718208727421,-6.54078339240215));
#80749=CARTESIAN_POINT('Ctrl Pts',(53.95,-6.47122943015123,-6.95508372791763));
#80750=CARTESIAN_POINT('Ctrl Pts',(54.1865412262364,-6.57965699823685,-6.53110589613718));
#80751=CARTESIAN_POINT('Ctrl Pts',(54.3836840636427,-6.68313474439608,-6.12648305687799));
#80752=CARTESIAN_POINT('',(30.5,-6.69861473382797,-6.06595258045412));
#80753=CARTESIAN_POINT('Origin',(54.35,0.,0.));
#80754=CARTESIAN_POINT('',(54.3836840636427,-5.39434373702554,-7.28691569216912));
#80755=CARTESIAN_POINT('Ctrl Pts',(54.3836840636427,-5.39434373702554,-7.28691569216912));
#80756=CARTESIAN_POINT('Ctrl Pts',(54.1865412262364,-5.80756637982325,-7.22629941152119));
#80757=CARTESIAN_POINT('Ctrl Pts',(53.95,-6.24055538374756,-7.16278357221404));
#80758=CARTESIAN_POINT('',(54.75,-4.77548435822936,-7.27219012019809));
#80759=CARTESIAN_POINT('Ctrl Pts',(54.3836840636385,-5.39434373702239,-7.28691569216838));
#80760=CARTESIAN_POINT('Ctrl Pts',(54.4264645321808,-5.33981558679448,-7.27405460498207));
#80761=CARTESIAN_POINT('Ctrl Pts',(54.4672398095033,-5.2842589712213,-7.26418094579635));
#80762=CARTESIAN_POINT('Ctrl Pts',(54.5981025051697,-5.09223784587415,-7.24122539887136));
#80763=CARTESIAN_POINT('Ctrl Pts',(54.687196533521,-4.93516659098831,-7.24246457082612));
#80764=CARTESIAN_POINT('Ctrl Pts',(54.75,-4.77548435822936,-7.27219012019808));
#80765=CARTESIAN_POINT('Origin',(54.75,0.,0.));
#80766=CARTESIAN_POINT('Origin',(41.725,-5.81744956039081,-7.22484963219258));
#80767=CARTESIAN_POINT('',(30.5,-5.39434373703405,-7.28691569217113));
#80768=CARTESIAN_POINT('',(30.5,-5.33252675337821,-7.29598372291775));
#80769=CARTESIAN_POINT('',(41.725,-5.39434373703405,-7.28691569217113));
#80770=CARTESIAN_POINT('Origin',(30.5,-5.05,-8.74685657822283));
#80771=CARTESIAN_POINT('',(30.5,-3.61348223613864,-8.31509655910253));
#80772=CARTESIAN_POINT('Origin',(30.5,-5.05,-8.74685657822283));
#80773=CARTESIAN_POINT('',(54.3836840636427,-3.61348223614116,-8.31509655909415));
#80774=CARTESIAN_POINT('',(41.725,-3.61348223613864,-8.31509655910253));
#80775=CARTESIAN_POINT('',(54.75,-3.91015920612708,-7.77178582970089));
#80776=CARTESIAN_POINT('Ctrl Pts',(54.75,-3.91015920612708,-7.77178582970089));
#80777=CARTESIAN_POINT('Ctrl Pts',(54.687196533521,-3.80457500885004,-7.89521192511717));
#80778=CARTESIAN_POINT('Ctrl Pts',(54.5981025051697,-3.72496622701464,-8.03062003607523));
#80779=CARTESIAN_POINT('Ctrl Pts',(54.4672398095032,-3.64883575113587,-8.20839298215164));
#80780=CARTESIAN_POINT('Ctrl Pts',(54.4264645321808,-3.62960828303242,-8.26144325217916));
#80781=CARTESIAN_POINT('Ctrl Pts',(54.3836840636385,-3.61348223614209,-8.31509655909106));
#80782=CARTESIAN_POINT('Origin',(54.75,-5.05,-8.74685657822283));
#80783=CARTESIAN_POINT('Origin',(41.725,-3.34817853980604,-8.65048392062934));
#80784=CARTESIAN_POINT('Ctrl Pts',(53.95,-3.08287484347344,-8.98587128215615));
#80785=CARTESIAN_POINT('Ctrl Pts',(54.1865412262364,-3.35437567581825,-8.64264972485195));
#80786=CARTESIAN_POINT('Ctrl Pts',(54.3836840636427,-3.61348223614116,-8.31509655909415));
#80787=CARTESIAN_POINT('',(30.5,-3.65224387295544,-8.26609549624456));
#80788=CARTESIAN_POINT('Origin',(54.35,0.,0.));
#80789=CARTESIAN_POINT('',(54.3836840636427,-1.96412259091325,-8.85100599400042));
#80790=CARTESIAN_POINT('Ctrl Pts',(54.3836840636427,-1.96412259091325,-8.85100599400042));
#80791=CARTESIAN_POINT('Ctrl Pts',(54.1865412262364,-2.36627512174265,-8.96370305672976));
#80792=CARTESIAN_POINT('Ctrl Pts',(53.95,-2.78766447874883,-9.08179094418728));
#80793=CARTESIAN_POINT('',(54.75,-1.40475584620536,-8.58584072834757));
#80794=CARTESIAN_POINT('Ctrl Pts',(54.3836840636385,-1.96412259091069,-8.85100599399847));
#80795=CARTESIAN_POINT('Ctrl Pts',(54.4264645321807,-1.91953972238479,-8.81707820944224));
#80796=CARTESIAN_POINT('Ctrl Pts',(54.4672398095032,-1.87280220757798,-8.78546126162393));
#80797=CARTESIAN_POINT('Ctrl Pts',(54.5981025051697,-1.70671904284191,-8.68638829807956));
#80798=CARTESIAN_POINT('Ctrl Pts',(54.687196533521,-1.56272329477366,-8.6236337030541));
#80799=CARTESIAN_POINT('Ctrl Pts',(54.75,-1.40475584620536,-8.58584072834756));
#80800=CARTESIAN_POINT('Origin',(54.75,0.,0.));
#80801=CARTESIAN_POINT('Origin',(41.725,-2.37589353483453,-8.9663984690965));
#80802=CARTESIAN_POINT('',(30.5,-1.96412259092022,-8.85100599400572));
#80803=CARTESIAN_POINT('',(30.5,-1.90396166591106,-8.83414681988681));
#80804=CARTESIAN_POINT('',(41.725,-1.96412259092022,-8.85100599400572));
#80805=CARTESIAN_POINT('Origin',(30.5,-1.05573747900331,-10.0446711432196));
#80806=CARTESIAN_POINT('',(30.5,0.0809741782038119,-9.06595432596881));
#80807=CARTESIAN_POINT('Origin',(30.5,-1.05573747900331,-10.0446711432196));
#80808=CARTESIAN_POINT('',(54.3836840636427,0.0809741781981025,-9.06595432596218));
#80809=CARTESIAN_POINT('',(41.725,0.0809741782038119,-9.06595432596881));
#80810=CARTESIAN_POINT('',(54.75,-0.411038102340181,-8.69028467188645));
#80811=CARTESIAN_POINT('Ctrl Pts',(54.75,-0.411038102340177,-8.69028467188645));
#80812=CARTESIAN_POINT('Ctrl Pts',(54.687196533521,-0.264380222801327,-8.76009505874624));
#80813=CARTESIAN_POINT('Ctrl Pts',(54.5981025051697,-0.136578541270819,
-8.85141671475685));
#80814=CARTESIAN_POINT('Ctrl Pts',(54.4672398095032,0.00527688047320916,
-8.98285532794201));
#80815=CARTESIAN_POINT('Ctrl Pts',(54.4264645321808,0.0444195353663464,
-9.02349864532112));
#80816=CARTESIAN_POINT('Ctrl Pts',(54.3836840636385,0.0809741781959984,
-9.06595432595973));
#80817=CARTESIAN_POINT('Origin',(54.75,-1.05573747900331,-10.0446711432196));
#80818=CARTESIAN_POINT('Origin',(41.725,0.459755494441719,-9.26443719180044));
#80819=CARTESIAN_POINT('Ctrl Pts',(53.95,0.838536810679625,-9.46292005763206));
#80820=CARTESIAN_POINT('Ctrl Pts',(54.1865412262364,0.450907674495762,-9.25980090013205));
#80821=CARTESIAN_POINT('Ctrl Pts',(54.3836840636427,0.0809741781981025,
-9.06595432596218));
#80822=CARTESIAN_POINT('',(30.5,0.025633133145034,-9.03695540561423));
#80823=CARTESIAN_POINT('Origin',(54.35,0.,0.));
#80824=CARTESIAN_POINT('',(54.3836840636427,1.8057131946615,-8.88467695060392));
#80825=CARTESIAN_POINT('Ctrl Pts',(54.3836840636427,1.8057131946615,-8.88467695060392));
#80826=CARTESIAN_POINT('Ctrl Pts',(54.1865412262364,1.48416660182181,-9.15120101074401));
#80827=CARTESIAN_POINT('Ctrl Pts',(53.95,1.14723893976231,-9.43047415642994));
#80828=CARTESIAN_POINT('',(54.75,2.20886771343379,-8.41492147465143));
#80829=CARTESIAN_POINT('Ctrl Pts',(54.3836840636385,1.80571319466305,-8.88467695060108));
#80830=CARTESIAN_POINT('Ctrl Pts',(54.4264645321808,1.83264199849617,-8.83554889084895));
#80831=CARTESIAN_POINT('Ctrl Pts',(54.4672398095032,1.8624790716295,-8.78765551190679));
#80832=CARTESIAN_POINT('Ctrl Pts',(54.5981025051697,1.97390698775344,-8.62959574718948));
#80833=CARTESIAN_POINT('Ctrl Pts',(54.687196533521,2.07992905600281,-8.5136982247713));
#80834=CARTESIAN_POINT('Ctrl Pts',(54.75,2.20886771343378,-8.41492147465143));
#80835=CARTESIAN_POINT('Origin',(54.75,0.,0.));
#80836=CARTESIAN_POINT('Origin',(41.725,1.4764760672098,-9.15757555352076));
#80837=CARTESIAN_POINT('',(30.5,1.8057131946573,-8.88467695061159));
#80838=CARTESIAN_POINT('',(30.5,1.85381569054083,-8.8448056759931));
#80839=CARTESIAN_POINT('',(41.725,1.8057131946573,-8.88467695061159));
#80840=CARTESIAN_POINT('Origin',(30.5,3.12107164318697,-9.60567081458105));
#80841=CARTESIAN_POINT('',(30.5,3.76142942150752,-8.24922622826565));
#80842=CARTESIAN_POINT('Origin',(30.5,3.12107164318697,-9.60567081458105));
#80843=CARTESIAN_POINT('',(54.3836840636427,3.76142942149961,-8.24922622826191));
#80844=CARTESIAN_POINT('',(41.725,3.76142942150752,-8.24922622826565));
#80845=CARTESIAN_POINT('',(54.75,3.15915522350527,-8.10615434554508));
#80846=CARTESIAN_POINT('Ctrl Pts',(54.75,3.15915522350528,-8.10615434554507));
#80847=CARTESIAN_POINT('Ctrl Pts',(54.687196533521,3.32152830558867,-8.11027817375286));
#80848=CARTESIAN_POINT('Ctrl Pts',(54.5981025051697,3.47542481503583,-8.1417230308606));
#80849=CARTESIAN_POINT('Ctrl Pts',(54.4672398095032,3.65847709150953,-8.20410038085247));
#80850=CARTESIAN_POINT('Ctrl Pts',(54.4264645321807,3.71076681256147,-8.22530914677538));
#80851=CARTESIAN_POINT('Ctrl Pts',(54.3836840636385,3.76142942149669,-8.24922622826054));
#80852=CARTESIAN_POINT('Origin',(54.75,3.12107164318697,-9.60567081458105));
#80853=CARTESIAN_POINT('Origin',(41.725,4.18819362695297,-8.27648510773958));
#80854=CARTESIAN_POINT('Ctrl Pts',(53.95,4.61495783239841,-8.30374398721351));
#80855=CARTESIAN_POINT('Ctrl Pts',(54.1865412262364,4.17822499152176,-8.27584837712898));
#80856=CARTESIAN_POINT('Ctrl Pts',(54.3836840636427,3.76142942149961,-8.24922622826191));
#80857=CARTESIAN_POINT('',(30.5,3.69907793765504,-8.2452436271907));
#80858=CARTESIAN_POINT('Origin',(54.35,0.,0.));
#80859=CARTESIAN_POINT('',(54.3836840636427,5.2633247644899,-7.38210654769183));
#80860=CARTESIAN_POINT('Ctrl Pts',(54.3836840636427,5.2633247644899,-7.38210654769183));
#80861=CARTESIAN_POINT('Ctrl Pts',(54.1865412262364,5.07798243670109,-7.75637317394928));
#80862=CARTESIAN_POINT('Ctrl Pts',(53.95,4.88377432324997,-8.14854271385775));
#80863=CARTESIAN_POINT('',(54.75,5.44055797848702,-6.78898585082642));
#80864=CARTESIAN_POINT('Ctrl Pts',(54.3836840636385,5.26332476449016,-7.38210654768861));
#80865=CARTESIAN_POINT('Ctrl Pts',(54.4264645321808,5.26794326880724,-7.32627290058613));
#80866=CARTESIAN_POINT('Ctrl Pts',(54.4672398095032,5.27572079926106,-7.2703842908369));
#80867=CARTESIAN_POINT('Ctrl Pts',(54.5981025051697,5.31322656778419,-7.08066769419416));
#80868=CARTESIAN_POINT('Ctrl Pts',(54.687196533521,5.3629427774341,-6.9316669789053));
#80869=CARTESIAN_POINT('Ctrl Pts',(54.75,5.44055797848701,-6.78898585082642));
#80870=CARTESIAN_POINT('Origin',(54.75,0.,0.));
#80871=CARTESIAN_POINT('Origin',(41.725,5.07354954386957,-7.76532463077915));
#80872=CARTESIAN_POINT('',(30.5,5.26332476448917,-7.38210654770055));
#80873=CARTESIAN_POINT('',(30.5,5.29105147271138,-7.32611727818317));
#80874=CARTESIAN_POINT('',(41.725,5.26332476448918,-7.38210654770055));
#80875=CARTESIAN_POINT('Origin',(30.5,6.75821912422446,-7.50576273732169));
#80876=CARTESIAN_POINT('',(30.5,6.79149934631904,-6.00613197382777));
#80877=CARTESIAN_POINT('Origin',(30.5,6.75821912422446,-7.50576273732169));
#80878=CARTESIAN_POINT('',(54.3836840636427,6.7914993463103,-6.00613197382758));
#80879=CARTESIAN_POINT('',(41.725,6.79149934631904,-6.00613197382777));
#80880=CARTESIAN_POINT('',(54.75,6.18310191118245,-6.12039629075862));
#80881=CARTESIAN_POINT('Ctrl Pts',(54.75,6.18310191118245,-6.12039629075862));
#80882=CARTESIAN_POINT('Ctrl Pts',(54.687196533521,6.33311441480502,-6.05812051295347));
#80883=CARTESIAN_POINT('Ctrl Pts',(54.5981025051697,6.48649564757952,-6.02425146969684));
#80884=CARTESIAN_POINT('Ctrl Pts',(54.4672398095032,6.67909337720287,-6.00678194600141));
#80885=CARTESIAN_POINT('Ctrl Pts',(54.4264645321807,6.73548879660653,-6.00488897216445));
#80886=CARTESIAN_POINT('Ctrl Pts',(54.3836840636385,6.79149934630707,-6.00613197382751));
#80887=CARTESIAN_POINT('Origin',(54.75,6.75821912422446,-7.50576273732169));
#80888=CARTESIAN_POINT('Origin',(41.725,7.19245503281942,-5.85745355904382));
#80889=CARTESIAN_POINT('Ctrl Pts',(53.95,7.5934107193198,-5.70877514425986));
#80890=CARTESIAN_POINT('Ctrl Pts',(54.1865412262364,7.18308924953126,-5.86092648599809));
#80891=CARTESIAN_POINT('Ctrl Pts',(54.3836840636427,6.7914993463103,-6.00613197382758));
#80892=CARTESIAN_POINT('',(30.5,6.7329185616764,-6.02785431993911));
#80893=CARTESIAN_POINT('Origin',(54.35,0.,0.));
#80894=CARTESIAN_POINT('',(54.3836840636427,7.81085966673361,-4.60310285835123));
#80895=CARTESIAN_POINT('Ctrl Pts',(54.3836840636427,7.81085966673361,-4.60310285835123));
#80896=CARTESIAN_POINT('Ctrl Pts',(54.1865412262364,7.7937689762525,-5.02039795094069));
#80897=CARTESIAN_POINT('Ctrl Pts',(53.95,7.77586075855085,-5.45765420887298));
#80898=CARTESIAN_POINT('',(54.75,7.73152634314226,-3.98917289739329));
#80899=CARTESIAN_POINT('Ctrl Pts',(54.3836840636385,7.81085966673255,-4.60310285834819));
#80900=CARTESIAN_POINT('Ctrl Pts',(54.4264645321807,7.79236929017938,-4.55021776871213));
#80901=CARTESIAN_POINT('Ctrl Pts',(54.4672398095032,7.77674247228156,-4.49599757651355));
#80902=CARTESIAN_POINT('Ctrl Pts',(54.5981025051697,7.73384100509704,-4.30742787102609));
#80903=CARTESIAN_POINT('Ctrl Pts',(54.687196533521,7.71865497184143,-4.15108754016899));
#80904=CARTESIAN_POINT('Ctrl Pts',(54.75,7.73152634314226,-3.98917289739329));
#80905=CARTESIAN_POINT('Origin',(54.75,0.,0.));
#80906=CARTESIAN_POINT('Origin',(41.725,7.79336021264368,-5.03037853361623));
#80907=CARTESIAN_POINT('',(30.5,7.8108596667365,-4.60310285835949));
#80908=CARTESIAN_POINT('',(30.5,7.81341638755651,-4.54067664728932));
#80909=CARTESIAN_POINT('',(41.725,7.8108596667365,-4.60310285835949));
#80910=CARTESIAN_POINT('Origin',(30.5,9.22680912219027,-4.10804009506559));
#80911=CARTESIAN_POINT('',(30.5,8.64725733531739,-2.72452293711905));
#80912=CARTESIAN_POINT('Origin',(30.5,9.22680912219027,-4.10804009506559));
#80913=CARTESIAN_POINT('',(54.3836840636427,8.64725733530932,-2.72452293712243));
#80914=CARTESIAN_POINT('',(41.725,8.64725733531739,-2.72452293711905));
#80915=CARTESIAN_POINT('',(54.75,8.13793410669875,-3.07636611524525));
#80916=CARTESIAN_POINT('Ctrl Pts',(54.75,8.13793410669875,-3.07636611524524));
#80917=CARTESIAN_POINT('Ctrl Pts',(54.687196533521,8.24964750716333,-2.95845877916736));
#80918=CARTESIAN_POINT('Ctrl Pts',(54.5981025051697,8.37599245469372,-2.86513210081603));
#80919=CARTESIAN_POINT('Ctrl Pts',(54.4672398095032,8.54483374031939,-2.77083634278586));
#80920=CARTESIAN_POINT('Ctrl Pts',(54.4264645321807,8.59558357772358,-2.74616894156258));
#80921=CARTESIAN_POINT('Ctrl Pts',(54.3836840636385,8.64725733530634,-2.72452293712368));
#80922=CARTESIAN_POINT('Origin',(54.75,9.22680912219027,-4.10804009506559));
#80923=CARTESIAN_POINT('Origin',(41.725,8.95307562210873,-2.42561507669435));
#80924=CARTESIAN_POINT('Ctrl Pts',(53.95,9.25889390890006,-2.12670721626965));
#80925=CARTESIAN_POINT('Ctrl Pts',(54.1865412262364,8.94593211997956,-2.43259716059258));
#80926=CARTESIAN_POINT('Ctrl Pts',(54.3836840636427,8.64725733530932,-2.72452293712243));
#80927=CARTESIAN_POINT('',(30.5,8.60257639973902,-2.7681942394327));
#80928=CARTESIAN_POINT('Origin',(54.5,-0.5,-1.73205080756888));
#80929=CARTESIAN_POINT('',(54.75,-2.,-1.15470053837925));
#80930=CARTESIAN_POINT('',(54.75,-5.55111512312578E-16,-2.3094010767585));
#80931=CARTESIAN_POINT('',(54.75,-0.625,-1.94855715851499));
#80932=CARTESIAN_POINT('',(54.25,-3.18172571617472E-16,-1.73205080756888));
#80933=CARTESIAN_POINT('',(54.75,-5.55111512312578E-16,-2.3094010767585));
#80934=CARTESIAN_POINT('',(54.25,-1.5,-0.866025403784439));
#80935=CARTESIAN_POINT('',(54.25,-0.375,-1.51554445662277));
#80936=CARTESIAN_POINT('',(54.75,-2.,-1.15470053837925));
#80937=CARTESIAN_POINT('Origin',(54.5,1.25,-1.29903810567666));
#80938=CARTESIAN_POINT('',(54.75,2.,-1.15470053837925));
#80939=CARTESIAN_POINT('',(54.75,1.375,-1.51554445662277));
#80940=CARTESIAN_POINT('',(54.25,1.5,-0.866025403784439));
#80941=CARTESIAN_POINT('',(54.75,2.,-1.15470053837925));
#80942=CARTESIAN_POINT('',(54.25,1.125,-1.08253175473055));
#80943=CARTESIAN_POINT('Origin',(54.5,0.5,1.73205080756888));
#80944=CARTESIAN_POINT('',(54.75,2.,1.15470053837925));
#80945=CARTESIAN_POINT('',(54.75,2.77555756156289E-16,2.3094010767585));
#80946=CARTESIAN_POINT('',(54.75,0.625,1.94855715851499));
#80947=CARTESIAN_POINT('',(54.25,1.06057523872491E-16,1.73205080756888));
#80948=CARTESIAN_POINT('',(54.75,0.,2.3094010767585));
#80949=CARTESIAN_POINT('',(54.25,1.5,0.866025403784439));
#80950=CARTESIAN_POINT('',(54.25,0.375,1.51554445662277));
#80951=CARTESIAN_POINT('',(54.25,1.5,0.866025403784439));
#80952=CARTESIAN_POINT('Origin',(54.5,-1.25,1.29903810567666));
#80953=CARTESIAN_POINT('',(54.25,-1.5,0.866025403784439));
#80954=CARTESIAN_POINT('',(54.25,-1.125,1.08253175473055));
#80955=CARTESIAN_POINT('',(54.75,-2.,1.15470053837925));
#80956=CARTESIAN_POINT('',(54.75,-1.375,1.51554445662277));
#80957=CARTESIAN_POINT('',(54.75,-2.,1.15470053837925));
#80958=CARTESIAN_POINT('Origin',(54.5,1.75,0.433012701892219));
#80959=CARTESIAN_POINT('',(54.75,2.,0.433012701892219));
#80960=CARTESIAN_POINT('',(54.25,1.5,0.433012701892219));
#80961=CARTESIAN_POINT('Origin',(54.5,-1.75,-0.43301270189222));
#80962=CARTESIAN_POINT('',(54.25,-1.5,-0.43301270189222));
#80963=CARTESIAN_POINT('',(54.75,-2.,-0.43301270189222));
#80964=CARTESIAN_POINT('Origin',(54.75,1.5,-0.866025403784439));
#80965=CARTESIAN_POINT('',(50.75,1.5,-0.866025403784439));
#80966=CARTESIAN_POINT('',(54.75,1.5,-0.866025403784439));
#80967=CARTESIAN_POINT('',(50.75,-2.77555756156289E-16,-1.73205080756888));
#80968=CARTESIAN_POINT('',(50.75,-3.18172571617472E-16,-1.73205080756888));
#80969=CARTESIAN_POINT('',(54.75,-3.18172571617472E-16,-1.73205080756888));
#80970=CARTESIAN_POINT('Origin',(54.75,1.5,0.866025403784439));
#80971=CARTESIAN_POINT('',(50.75,1.5,0.866025403784439));
#80972=CARTESIAN_POINT('',(54.75,1.5,0.866025403784439));
#80973=CARTESIAN_POINT('',(50.75,1.5,-0.866025403784439));
#80974=CARTESIAN_POINT('Origin',(54.75,0.,1.73205080756888));
#80975=CARTESIAN_POINT('',(50.75,0.,1.73205080756888));
#80976=CARTESIAN_POINT('',(54.75,1.06057523872491E-16,1.73205080756888));
#80977=CARTESIAN_POINT('',(50.75,1.5,0.866025403784439));
#80978=CARTESIAN_POINT('Origin',(54.75,0.,0.));
#80979=CARTESIAN_POINT('Origin',(54.75,0.,0.));
#80980=CARTESIAN_POINT('Origin',(54.75,-1.5,0.866025403784439));
#80981=CARTESIAN_POINT('',(50.75,-1.5,0.866025403784439));
#80982=CARTESIAN_POINT('',(54.75,-1.5,0.866025403784439));
#80983=CARTESIAN_POINT('',(50.75,1.06057523872491E-16,1.73205080756888));
#80984=CARTESIAN_POINT('Origin',(54.75,-1.5,-0.866025403784439));
#80985=CARTESIAN_POINT('',(50.75,-1.5,-0.866025403784439));
#80986=CARTESIAN_POINT('',(54.75,-1.5,-0.866025403784439));
#80987=CARTESIAN_POINT('',(50.75,-1.5,0.866025403784439));
#80988=CARTESIAN_POINT('Origin',(54.75,-2.77555756156289E-16,-1.73205080756888));
#80989=CARTESIAN_POINT('',(50.75,-1.5,-0.866025403784439));
#80990=CARTESIAN_POINT('Origin',(50.75,0.,0.));
#80991=CARTESIAN_POINT('Origin',(30.5,9.22680912219027,-4.10804009506559));
#80992=CARTESIAN_POINT('Origin',(30.5,6.75821912422446,-7.50576273732169));
#80993=CARTESIAN_POINT('Origin',(30.5,3.12107164318697,-9.60567081458105));
#80994=CARTESIAN_POINT('Origin',(30.5,-1.05573747900331,-10.0446711432196));
#80995=CARTESIAN_POINT('Origin',(30.5,-5.05,-8.74685657822283));
#80996=CARTESIAN_POINT('Origin',(30.5,-8.17107164318697,-5.93663104815398));
#80997=CARTESIAN_POINT('Origin',(30.5,-9.87929076741144,-2.09990807725937));
#80998=CARTESIAN_POINT('Origin',(30.5,-9.87929076741144,2.09990807725937));
#80999=CARTESIAN_POINT('Origin',(30.5,-8.17107164318697,5.93663104815398));
#81000=CARTESIAN_POINT('Origin',(30.5,-5.05,8.74685657822283));
#81001=CARTESIAN_POINT('Origin',(30.5,-1.0557374790033,10.0446711432196));
#81002=CARTESIAN_POINT('Origin',(30.5,3.12107164318697,9.60567081458105));
#81003=CARTESIAN_POINT('Origin',(30.5,6.75821912422447,7.50576273732168));
#81004=CARTESIAN_POINT('Origin',(30.5,9.22680912219027,4.10804009506558));
#81005=CARTESIAN_POINT('Origin',(30.5,10.1,0.));
#81006=CARTESIAN_POINT('Origin',(54.35,0.,0.));
#81007=CARTESIAN_POINT('Origin',(27.2,0.,0.));
#81008=CARTESIAN_POINT('',(27.4,-8.,-9.79717439317883E-16));
#81009=CARTESIAN_POINT('Origin',(27.4,0.,0.));
#81010=CARTESIAN_POINT('',(27.2,-7.8,-9.55224503334935E-16));
#81011=CARTESIAN_POINT('Origin',(28.2,0.,0.));
#81012=CARTESIAN_POINT('',(29.,-8.,-9.79717439317883E-16));
#81013=CARTESIAN_POINT('Origin',(29.,0.,0.));
#81014=CARTESIAN_POINT('',(28.2,-8.,-9.79717439317883E-16));
#81015=CARTESIAN_POINT('Origin',(29.,9.,0.));
#81016=CARTESIAN_POINT('',(29.,-9.,-1.10218211923262E-15));
#81017=CARTESIAN_POINT('Origin',(29.,0.,0.));
#81018=CARTESIAN_POINT('Origin',(29.25,0.,0.));
#81019=CARTESIAN_POINT('',(29.25,-9.25,-1.1327982892113E-15));
#81020=CARTESIAN_POINT('Origin',(49.,5.05,0.));
#82361=UNCERTAINTY_MEASURE_WITH_UNIT(LENGTH_MEASURE(0.01),#82385,
'DISTANCE_ACCURACY_VALUE',
'Maximum model space distance between geometric entities at asserted c
onnectivities');
#82363=UNCERTAINTY_MEASURE_WITH_UNIT(LENGTH_MEASURE(0.01),#82385,
'DISTANCE_ACCURACY_VALUE',
'Maximum model space distance between geometric entities at asserted c
onnectivities');
#82382=(
GEOMETRIC_REPRESENTATION_CONTEXT(3)
GLOBAL_UNCERTAINTY_ASSIGNED_CONTEXT((#82361))
GLOBAL_UNIT_ASSIGNED_CONTEXT((#82385,#82387,#82388))
REPRESENTATION_CONTEXT('','3D')
);
#82384=(
GEOMETRIC_REPRESENTATION_CONTEXT(3)
GLOBAL_UNCERTAINTY_ASSIGNED_CONTEXT((#82363))
GLOBAL_UNIT_ASSIGNED_CONTEXT((#82385,#82387,#82388))
REPRESENTATION_CONTEXT('','3D')
);
#82385=(
LENGTH_UNIT()
NAMED_UNIT(*)
SI_UNIT(.MILLI.,.METRE.)
);
#82387=(
NAMED_UNIT(*)
PLANE_ANGLE_UNIT()
SI_UNIT($,.RADIAN.)
);
#82388=(
NAMED_UNIT(*)
SI_UNIT($,.STERADIAN.)
SOLID_ANGLE_UNIT()
);
#82407=SHAPE_DEFINITION_REPRESENTATION(#82427,#82483);
#82427=PRODUCT_DEFINITION_SHAPE('',$,#82504);
#82483=SHAPE_REPRESENTATION('',(#33154),#82382);
#82485=PRODUCT_DEFINITION_CONTEXT('part definition',#82547,'design');
#82504=PRODUCT_DEFINITION('2026-10-20-12-38-15-744',
'06_AJS_Fluted_Knob',#82524,#82485);
#82524=PRODUCT_DEFINITION_FORMATION('',$,#82567);
#82547=APPLICATION_CONTEXT(
'Core Data for Automotive Mechanical Design Process');
#82548=PRODUCT_CONTEXT('part definition',#82547,'mechanical');
#82567=PRODUCT('2026-10-20-12-38-15-744','06_AJS_Fluted_Knob',$,(#82548));
#82618=COLOUR_RGB('Sky Blue',0.24,0.69,0.87);
#82619=FILL_AREA_STYLE_COLOUR('',#82618);
#82620=FILL_AREA_STYLE('',(#82619));
#82621=SURFACE_STYLE_FILL_AREA(#82620);
#82622=SURFACE_SIDE_STYLE('',(#82621));
#82623=SURFACE_STYLE_USAGE(.BOTH.,#82622);
#82624=PRESENTATION_STYLE_ASSIGNMENT((#82623));
ENDSEC;
END-ISO-10303-21;
